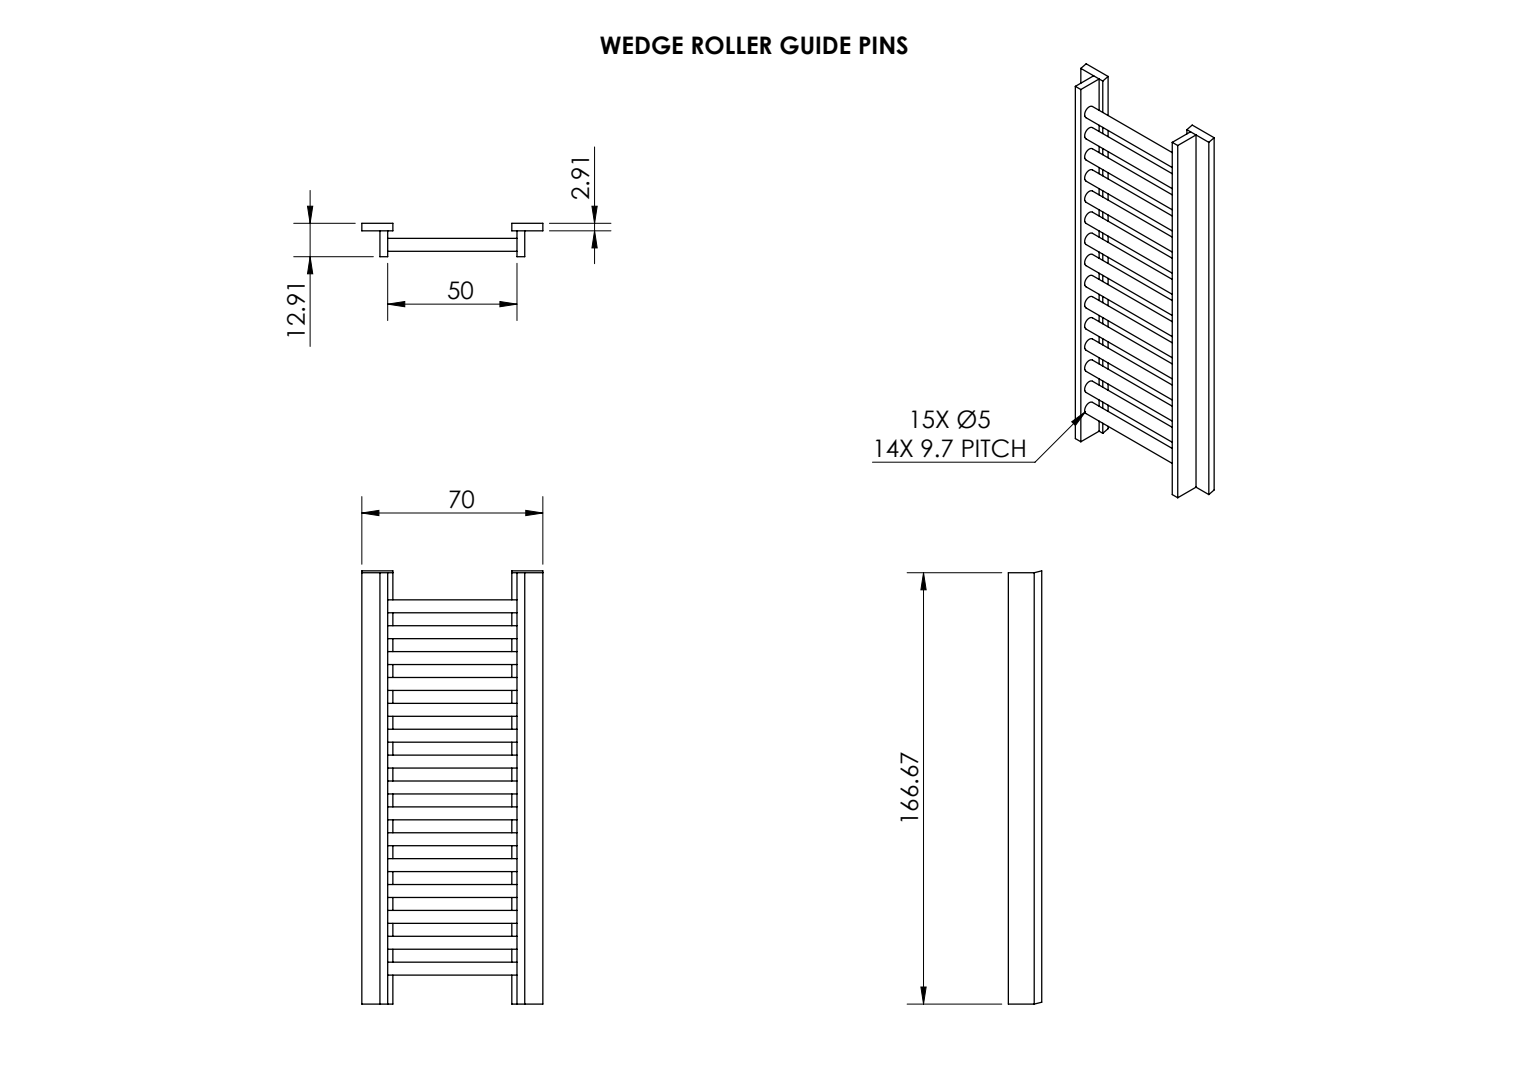
ISO-10303-21;
HEADER;
FILE_DESCRIPTION (('STEP AP214'),
    '1' );
FILE_NAME ('Wedge Roller Guide Pins.step',
    '2026-09-24T10:26:00',
    ( '' ),
    ( '' ),
    'SwSTEP 2.0',
    'SolidWorks 2026',
    '' );
FILE_SCHEMA (( 'AUTOMOTIVE_DESIGN' ));
ENDSEC;

DATA;
#3=CARTESIAN_POINT ( 'NONE',  ( 34.85300976710104948, 100.8957249956400375, 25.00000000000000000 ) ) ;
#7=CARTESIAN_POINT ( 'NONE',  ( 59.10657227073432551, 3.881474981106830313, 25.00000000000000000 ) ) ;
#45=VERTEX_POINT ( 'NONE', #1089 ) ;
#50=CIRCLE ( 'NONE', #10087, 2.500000000000002220 ) ;
#51=CIRCLE ( 'NONE', #7981, 2.500000000000002220 ) ;
#55=VERTEX_POINT ( 'NONE', #5546 ) ;
#59=MECHANICAL_DESIGN_GEOMETRIC_PRESENTATION_REPRESENTATION('',(#3339),#8217);
#68=DIRECTION ( 'NONE',  ( -1.000000000000000000, 0.000000000000000000, 0.000000000000000000 ) ) ;
#75=EDGE_CURVE ( 'NONE', #7740, #14384, #13409, .T. ) ;
#106=LINE ( 'NONE', #11351, #1126 ) ;
#108=( NAMED_UNIT ( * ) PLANE_ANGLE_UNIT ( ) SI_UNIT ( $, .RADIAN. ) );
#114=CYLINDRICAL_SURFACE ( 'NONE', #8701, 2.500000000000002220 ) ;
#138=AXIS2_PLACEMENT_3D ( 'NONE', #9240, #11510, #4853 ) ;
#139=FACE_OUTER_BOUND ( 'NONE', #10085, .T. ) ;
#141=EDGE_CURVE ( 'NONE', #4176, #9400, #11330, .T. ) ;
#150=EDGE_CURVE ( 'NONE', #7089, #2949, #9184, .T. ) ;
#158=ORIENTED_EDGE ( 'NONE', *, *, #2244, .F. ) ;
#159=CARTESIAN_POINT ( 'NONE',  ( 56.68121602037099649, 13.58289998256015352, 25.00000000000000000 ) ) ;
#167=CARTESIAN_POINT ( 'NONE',  ( 0.000000000000000000, 0.000000000000000000, 0.000000000000000000 ) ) ;
#174=LINE ( 'NONE', #1203, #523 ) ;
#175=AXIS2_PLACEMENT_3D ( 'NONE', #2230, #7697, #10922 ) ;
#184=DIRECTION ( 'NONE',  ( -1.000000000000000000, 0.000000000000000000, 0.000000000000000000 ) ) ;
#187=AXIS2_PLACEMENT_3D ( 'NONE', #14289, #6433, #6375 ) ;
#192=VERTEX_POINT ( 'NONE', #361 ) ;
#207=ORIENTED_EDGE ( 'NONE', *, *, #6472, .T. ) ;
#217=CARTESIAN_POINT ( 'NONE',  ( 56.75585977000769589, 23.28432498401347672, 25.00000000000000000 ) ) ;
#219=CARTESIAN_POINT ( 'NONE',  ( 62.10586122665984732, -20.42344490663941414, -23.00000000000000000 ) ) ;
#245=ORIENTED_EDGE ( 'NONE', *, *, #3357, .T. ) ;
#255=DIRECTION ( 'NONE',  ( 0.000000000000000000, 0.000000000000000000, 1.000000000000000000 ) ) ;
#257=FACE_OUTER_BOUND ( 'NONE', #7644, .T. ) ;
#260=VERTEX_POINT ( 'NONE', #11845 ) ;
#262=VECTOR ( 'NONE', #2943, 1000.000000000000114 ) ;
#271=CARTESIAN_POINT ( 'NONE',  ( 66.53192852109765454, -5.819950020346492892, -25.00000000000000000 ) ) ;
#280=CYLINDRICAL_SURFACE ( 'NONE', #1408, 2.500000000000002220 ) ;
#290=DIRECTION ( 'NONE',  ( -1.000000000000000000, 0.000000000000000000, 0.000000000000000000 ) ) ;
#293=EDGE_CURVE ( 'NONE', #3067, #10101, #2628, .T. ) ;
#296=CARTESIAN_POINT ( 'NONE',  ( 61.53192852109764743, -5.819950020346492892, -25.00000000000000000 ) ) ;
#304=CARTESIAN_POINT ( 'NONE',  ( 63.34848382498275754, 15.83712095624566984, 0.000000000000000000 ) ) ;
#318=DIRECTION ( 'NONE',  ( 0.000000000000000000, 0.000000000000000000, -1.000000000000000000 ) ) ;
#319=AXIS2_PLACEMENT_3D ( 'NONE', #14262, #4250, #9862 ) ;
#332=EDGE_LOOP ( 'NONE', ( #2235, #9839 ) ) ;
#356=EDGE_CURVE ( 'NONE', #7502, #4025, #7084, .T. ) ;
#361=CARTESIAN_POINT ( 'NONE',  ( 35.00229726637439143, 120.2985749985466839, 25.00000000000000000 ) ) ;
#367=EDGE_CURVE ( 'NONE', #6880, #5464, #10123, .T. ) ;
#370=ADVANCED_FACE ( 'NONE', ( #3209 ), #923, .F. ) ;
#385=CARTESIAN_POINT ( 'NONE',  ( 54.33050351964436686, 32.98574998546678927, 25.00000000000000000 ) ) ;
#403=ORIENTED_EDGE ( 'NONE', *, *, #3357, .F. ) ;
#418=EDGE_CURVE ( 'NONE', #12547, #7049, #5258, .T. ) ;
#436=VECTOR ( 'NONE', #12555, 999.9999999999998863 ) ;
#450=ORIENTED_EDGE ( 'NONE', *, *, #2914, .T. ) ;
#453=DIRECTION ( 'NONE',  ( 0.000000000000000000, 0.000000000000000000, -1.000000000000000000 ) ) ;
#461=CARTESIAN_POINT ( 'NONE',  ( 63.34848382498275754, 15.83712095624566984, 0.000000000000000000 ) ) ;
#474=ORIENTED_EDGE ( 'NONE', *, *, #4676, .T. ) ;
#482=PLANE ( 'NONE',  #7880 ) ;
#483=DIRECTION ( 'NONE',  ( 0.000000000000000000, 0.000000000000000000, -1.000000000000000000 ) ) ;
#490=DIRECTION ( 'NONE',  ( 1.000000000000000000, 0.000000000000000000, 0.000000000000000000 ) ) ;
#494=CARTESIAN_POINT ( 'NONE',  ( 49.55443476855437268, 62.09002498982675888, 25.00000000000000000 ) ) ;
#516=ORIENTED_EDGE ( 'NONE', *, *, #14434, .F. ) ;
#523=VECTOR ( 'NONE', #2168, 1000.000000000000000 ) ;
#536=CARTESIAN_POINT ( 'NONE',  ( 37.35300976710104948, 100.8957249956400375, -25.00000000000000000 ) ) ;
#544=LINE ( 'NONE', #5067, #7395 ) ;
#552=APPLICATION_CONTEXT ( 'automotive_design' ) ;
#554=AXIS2_PLACEMENT_3D ( 'NONE', #7102, #318, #1552 ) ;
#556=EDGE_CURVE ( 'NONE', #7883, #4518, #5673, .T. ) ;
#558=ORIENTED_EDGE ( 'NONE', *, *, #7367, .T. ) ;
#561=AXIS2_PLACEMENT_3D ( 'NONE', #10302, #7885, #290 ) ;
#563=CARTESIAN_POINT ( 'NONE',  ( 61.60657227073433262, 3.881474981106830313, 25.00000000000000000 ) ) ;
#564=FACE_BOUND ( 'NONE', #13096, .T. ) ;
#566=DIRECTION ( 'NONE',  ( 0.000000000000000000, 0.000000000000000000, 1.000000000000000000 ) ) ;
#581=CARTESIAN_POINT ( 'NONE',  ( 0.000000000000000000, 0.000000000000000000, 35.00000000000000000 ) ) ;
#591=CARTESIAN_POINT ( 'NONE',  ( 30.00229726637438432, 120.2985749985466839, -25.00000000000000000 ) ) ;
#596=DIRECTION ( 'NONE',  ( -1.000000000000000000, 0.000000000000000000, 0.000000000000000000 ) ) ;
#614=CARTESIAN_POINT ( 'NONE',  ( 54.25585977000769589, 23.28432498401347672, 25.00000000000000000 ) ) ;
#635=DIRECTION ( 'NONE',  ( 0.000000000000000000, 0.000000000000000000, 1.000000000000000000 ) ) ;
#648=DIRECTION ( 'NONE',  ( 0.000000000000000000, 0.000000000000000000, -1.000000000000000000 ) ) ;
#666=AXIS2_PLACEMENT_3D ( 'NONE', #7553, #831, #14236 ) ;
#674=EDGE_CURVE ( 'NONE', #2739, #5618, #12700, .T. ) ;
#677=VECTOR ( 'NONE', #3560, 999.9999999999998863 ) ;
#680=ORIENTED_EDGE ( 'NONE', *, *, #3167, .T. ) ;
#684=CARTESIAN_POINT ( 'NONE',  ( 62.10586122665984732, -20.42344490663941414, 35.00000000000000000 ) ) ;
#685=EDGE_CURVE ( 'NONE', #3184, #7164, #14140, .T. ) ;
#689=CARTESIAN_POINT ( 'NONE',  ( 64.03192852109765454, -5.819950020346492892, 25.00000000000000000 ) ) ;
#696=VERTEX_POINT ( 'NONE', #8297 ) ;
#707=FACE_BOUND ( 'NONE', #8200, .T. ) ;
#727=DIRECTION ( 'NONE',  ( -0.9701425001453319874, -0.2425356250363328026, 0.000000000000000000 ) ) ;
#729=DIRECTION ( 'NONE',  ( 0.000000000000000000, 0.000000000000000000, -1.000000000000000000 ) ) ;
#778=CARTESIAN_POINT ( 'NONE',  ( 71.80728622811317052, -17.99808865627607801, 28.00000000000000000 ) ) ;
#788=PLANE ( 'NONE',  #1131 ) ;
#793=CYLINDRICAL_SURFACE ( 'NONE', #14229, 2.500000000000002220 ) ;
#812=LINE ( 'NONE', #2952, #993 ) ;
#828=CARTESIAN_POINT ( 'NONE',  ( 51.90514726928103073, 42.68717498692012668, 25.00000000000000000 ) ) ;
#829=ORIENTED_EDGE ( 'NONE', *, *, #5080, .F. ) ;
#830=ORIENTED_EDGE ( 'NONE', *, *, #13086, .T. ) ;
#831=DIRECTION ( 'NONE',  ( 0.000000000000000000, 0.000000000000000000, -1.000000000000000000 ) ) ;
#833=ORIENTED_EDGE ( 'NONE', *, *, #2397, .F. ) ;
#848=DIRECTION ( 'NONE',  ( -1.000000000000000000, 0.000000000000000000, 0.000000000000000000 ) ) ;
#852=SHAPE_REPRESENTATION ( 'Wedge Roller Guide Pins', ( #11025 ), #12660 ) ;
#861=DIRECTION ( 'NONE',  ( 0.000000000000000000, 0.000000000000000000, -1.000000000000000000 ) ) ;
#877=ORIENTED_EDGE ( 'NONE', *, *, #367, .F. ) ;
#884=CIRCLE ( 'NONE', #1928, 2.500000000000002220 ) ;
#896=CARTESIAN_POINT ( 'NONE',  ( 66.53192852109765454, -5.819950020346492892, 25.00000000000000000 ) ) ;
#899=ORIENTED_EDGE ( 'NONE', *, *, #1154, .F. ) ;
#901=FACE_BOUND ( 'NONE', #9182, .T. ) ;
#903=EDGE_LOOP ( 'NONE', ( #2586, #3281, #10639, #10466 ) ) ;
#908=VERTEX_POINT ( 'NONE', #4230 ) ;
#911=CARTESIAN_POINT ( 'NONE',  ( 61.60657227073433262, 3.881474981106830313, 25.00000000000000000 ) ) ;
#921=ORIENTED_EDGE ( 'NONE', *, *, #4211, .T. ) ;
#922=VECTOR ( 'NONE', #9203, 1000.000000000000114 ) ;
#923=PLANE ( 'NONE',  #8498 ) ;
#945=VECTOR ( 'NONE', #3041, 1000.000000000000000 ) ;
#952=CARTESIAN_POINT ( 'NONE',  ( 47.05443476855437268, 62.09002498982675888, 25.00000000000000000 ) ) ;
#956=DIRECTION ( 'NONE',  ( 1.000000000000000000, 0.000000000000000000, 0.000000000000000000 ) ) ;
#958=DIRECTION ( 'NONE',  ( 0.000000000000000000, 0.000000000000000000, -1.000000000000000000 ) ) ;
#971=ORIENTED_EDGE ( 'NONE', *, *, #11807, .T. ) ;
#979=AXIS2_PLACEMENT_3D ( 'NONE', #13212, #11893, #4294 ) ;
#992=VERTEX_POINT ( 'NONE', #4519 ) ;
#993=VECTOR ( 'NONE', #12897, 999.9999999999998863 ) ;
#1038=CARTESIAN_POINT ( 'NONE',  ( 18.68170757442808849, 141.2731697022877313, 35.00000000000000000 ) ) ;
#1050=CARTESIAN_POINT ( 'NONE',  ( 31.38313257588138683, 143.6985259526510390, -28.00000000000000000 ) ) ;
#1054=PRESENTATION_STYLE_ASSIGNMENT (( #2158 ) ) ;
#1055=EDGE_LOOP ( 'NONE', ( #1751, #5944 ) ) ;
#1058=DIRECTION ( 'NONE',  ( -1.000000000000000000, 0.000000000000000000, 0.000000000000000000 ) ) ;
#1087=ORIENTED_EDGE ( 'NONE', *, *, #7522, .T. ) ;
#1089=CARTESIAN_POINT ( 'NONE',  ( 62.10586122665987574, -20.42344490663940704, -28.00000000000000000 ) ) ;
#1090=ORIENTED_EDGE ( 'NONE', *, *, #9852, .F. ) ;
#1094=CARTESIAN_POINT ( 'NONE',  ( 27.57694101601105530, 130.0000000000000000, 25.00000000000000000 ) ) ;
#1095=CARTESIAN_POINT ( 'NONE',  ( 42.20372226782770753, 81.49287499273339108, 25.00000000000000000 ) ) ;
#1112=FACE_OUTER_BOUND ( 'NONE', #2519, .T. ) ;
#1114=CARTESIAN_POINT ( 'NONE',  ( 47.05443476855437268, 62.09002498982675888, 25.00000000000000000 ) ) ;
#1121=CARTESIAN_POINT ( 'NONE',  ( 54.40514726928103784, 42.68717498692012668, 25.00000000000000000 ) ) ;
#1125=LINE ( 'NONE', #8872, #7058 ) ;
#1126=VECTOR ( 'NONE', #6747, 1000.000000000000000 ) ;
#1131=AXIS2_PLACEMENT_3D ( 'NONE', #7566, #1881, #14324 ) ;
#1147=EDGE_LOOP ( 'NONE', ( #6680, #4247, #9054, #1407 ) ) ;
#1149=ORIENTED_EDGE ( 'NONE', *, *, #1431, .F. ) ;
#1154=EDGE_CURVE ( 'NONE', #13574, #3245, #13934, .T. ) ;
#1159=AXIS2_PLACEMENT_3D ( 'NONE', #13106, #727, #3082 ) ;
#1176=VERTEX_POINT ( 'NONE', #5217 ) ;
#1180=DIRECTION ( 'NONE',  ( 0.000000000000000000, 0.000000000000000000, -1.000000000000000000 ) ) ;
#1193=DIRECTION ( 'NONE',  ( -0.000000000000000000, -0.000000000000000000, -1.000000000000000000 ) ) ;
#1195=ORIENTED_EDGE ( 'NONE', *, *, #13325, .F. ) ;
#1197=ORIENTED_EDGE ( 'NONE', *, *, #11455, .F. ) ;
#1198=EDGE_CURVE ( 'NONE', #11002, #6663, #1854, .T. ) ;
#1199=CIRCLE ( 'NONE', #6095, 2.500000000000002220 ) ;
#1203=CARTESIAN_POINT ( 'NONE',  ( 44.70372226782771463, 81.49287499273339108, 25.00000000000000000 ) ) ;
#1207=DIRECTION ( 'NONE',  ( 0.000000000000000000, 0.000000000000000000, -1.000000000000000000 ) ) ;
#1208=ORIENTED_EDGE ( 'NONE', *, *, #13188, .T. ) ;
#1210=VERTEX_POINT ( 'NONE', #11953 ) ;
#1218=ADVANCED_FACE ( 'NONE', ( #8573 ), #10705, .T. ) ;
#1221=ORIENTED_EDGE ( 'NONE', *, *, #3777, .T. ) ;
#1242=VECTOR ( 'NONE', #3558, 1000.000000000000000 ) ;
#1251=ORIENTED_EDGE ( 'NONE', *, *, #10457, .T. ) ;
#1266=EDGE_CURVE ( 'NONE', #9400, #6663, #2842, .T. ) ;
#1275=CARTESIAN_POINT ( 'NONE',  ( 42.20372226782770753, 81.49287499273339108, 25.00000000000000000 ) ) ;
#1280=ORIENTED_EDGE ( 'NONE', *, *, #13856, .T. ) ;
#1292=CYLINDRICAL_SURFACE ( 'NONE', #4914, 2.500000000000002220 ) ;
#1300=CARTESIAN_POINT ( 'NONE',  ( 56.68121602037099649, 13.58289998256015352, 25.00000000000000000 ) ) ;
#1312=DIRECTION ( 'NONE',  ( -0.000000000000000000, -0.000000000000000000, -1.000000000000000000 ) ) ;
#1328=VERTEX_POINT ( 'NONE', #7687 ) ;
#1349=AXIS2_PLACEMENT_3D ( 'NONE', #1038, #4350, #9963 ) ;
#1351=AXIS2_PLACEMENT_3D ( 'NONE', #12401, #11364, #7926 ) ;
#1378=LINE ( 'NONE', #10313, #262 ) ;
#1385=ORIENTED_EDGE ( 'NONE', *, *, #13324, .T. ) ;
#1389=AXIS2_PLACEMENT_3D ( 'NONE', #2479, #13763, #7222 ) ;
#1407=ORIENTED_EDGE ( 'NONE', *, *, #10352, .T. ) ;
#1408=AXIS2_PLACEMENT_3D ( 'NONE', #4546, #5891, #4746 ) ;
#1409=DIRECTION ( 'NONE',  ( 0.000000000000000000, 0.000000000000000000, 1.000000000000000000 ) ) ;
#1421=CARTESIAN_POINT ( 'NONE',  ( 21.68170757442808849, 141.2731697022877313, 35.00000000000000000 ) ) ;
#1425=AXIS2_PLACEMENT_3D ( 'NONE', #7083, #3889, #12576 ) ;
#1431=EDGE_CURVE ( 'NONE', #4518, #7883, #10070, .T. ) ;
#1439=AXIS2_PLACEMENT_3D ( 'NONE', #11177, #2196, #10158 ) ;
#1449=AXIS2_PLACEMENT_3D ( 'NONE', #4221, #13074, #9757 ) ;
#1452=ORIENTED_EDGE ( 'NONE', *, *, #11500, .F. ) ;
#1453=EDGE_CURVE ( 'NONE', #7600, #3428, #1733, .T. ) ;
#1457=CARTESIAN_POINT ( 'NONE',  ( 37.27836601746437850, 91.19429999418670718, 25.00000000000000000 ) ) ;
#1459=ADVANCED_FACE ( 'NONE', ( #12163 ), #10983, .T. ) ;
#1480=FACE_OUTER_BOUND ( 'NONE', #4601, .T. ) ;
#1481=ADVANCED_FACE ( 'NONE', ( #1112 ), #5566, .T. ) ;
#1484=VERTEX_POINT ( 'NONE', #11203 ) ;
#1508=ORIENTED_EDGE ( 'NONE', *, *, #9688, .F. ) ;
#1532=CARTESIAN_POINT ( 'NONE',  ( 51.90514726928103073, 42.68717498692012668, 25.00000000000000000 ) ) ;
#1549=PLANE ( 'NONE',  #5866 ) ;
#1552=DIRECTION ( 'NONE',  ( -1.000000000000000000, 0.000000000000000000, 0.000000000000000000 ) ) ;
#1567=ORIENTED_EDGE ( 'NONE', *, *, #556, .T. ) ;
#1569=FACE_BOUND ( 'NONE', #11379, .T. ) ;
#1576=ADVANCED_FACE ( 'NONE', ( #4836 ), #8046, .T. ) ;
#1587=AXIS2_PLACEMENT_3D ( 'NONE', #581, #9640, #10739 ) ;
#1595=AXIS2_PLACEMENT_3D ( 'NONE', #2769, #12950, #6194 ) ;
#1609=ORIENTED_EDGE ( 'NONE', *, *, #9227, .F. ) ;
#1638=DIRECTION ( 'NONE',  ( -1.000000000000000000, 0.000000000000000000, 0.000000000000000000 ) ) ;
#1640=LINE ( 'NONE', #6011, #3763 ) ;
#1646=LINE ( 'NONE', #778, #12787 ) ;
#1648=FACE_BOUND ( 'NONE', #6730, .T. ) ;
#1676=LINE ( 'NONE', #2631, #9345 ) ;
#1679=LINE ( 'NONE', #7224, #8428 ) ;
#1689=VECTOR ( 'NONE', #13552, 1000.000000000000000 ) ;
#1700=CIRCLE ( 'NONE', #7988, 2.500000000000002220 ) ;
#1702=VERTEX_POINT ( 'NONE', #11867 ) ;
#1703=ORIENTED_EDGE ( 'NONE', *, *, #2205, .F. ) ;
#1719=DIRECTION ( 'NONE',  ( 0.000000000000000000, 0.000000000000000000, 1.000000000000000000 ) ) ;
#1725=PLANE ( 'NONE',  #4726 ) ;
#1733=LINE ( 'NONE', #10655, #7488 ) ;
#1735=ORIENTED_EDGE ( 'NONE', *, *, #13842, .F. ) ;
#1751=ORIENTED_EDGE ( 'NONE', *, *, #13733, .F. ) ;
#1781=VERTEX_POINT ( 'NONE', #10624 ) ;
#1786=CARTESIAN_POINT ( 'NONE',  ( 44.70372226782771463, 81.49287499273339108, -25.00000000000000000 ) ) ;
#1789=CARTESIAN_POINT ( 'NONE',  ( 21.68170757442808849, 141.2731697022877313, -35.00000000000000000 ) ) ;
#1801=FACE_OUTER_BOUND ( 'NONE', #11405, .T. ) ;
#1813=AXIS2_PLACEMENT_3D ( 'NONE', #8430, #7399, #9537 ) ;
#1819=EDGE_CURVE ( 'NONE', #4025, #7502, #11428, .T. ) ;
#1842=CARTESIAN_POINT ( 'NONE',  ( 62.10586122665984732, -20.42344490663941414, -35.00000000000000000 ) ) ;
#1846=EDGE_LOOP ( 'NONE', ( #9526, #2877, #13120, #11097 ) ) ;
#1849=DIRECTION ( 'NONE',  ( 1.000000000000000000, 0.000000000000000000, 0.000000000000000000 ) ) ;
#1851=EDGE_CURVE ( 'NONE', #8043, #3245, #6575, .T. ) ;
#1854=LINE ( 'NONE', #10984, #945 ) ;
#1881=DIRECTION ( 'NONE',  ( 0.9701425001453319874, 0.2425356250363328026, 0.000000000000000000 ) ) ;
#1897=CARTESIAN_POINT ( 'NONE',  ( 31.38313257588138683, 143.6985259526510390, -28.00000000000000000 ) ) ;
#1911=ADVANCED_FACE ( 'NONE', ( #13331 ), #6651, .T. ) ;
#1917=DIRECTION ( 'NONE',  ( 0.000000000000000000, 0.000000000000000000, -1.000000000000000000 ) ) ;
#1925=FACE_OUTER_BOUND ( 'NONE', #13791, .T. ) ;
#1928=AXIS2_PLACEMENT_3D ( 'NONE', #11960, #10917, #1936 ) ;
#1931=CARTESIAN_POINT ( 'NONE',  ( 59.18121602037099649, 13.58289998256015352, -25.00000000000000000 ) ) ;
#1932=CARTESIAN_POINT ( 'NONE',  ( 54.25585977000769589, 23.28432498401347672, 25.00000000000000000 ) ) ;
#1935=CARTESIAN_POINT ( 'NONE',  ( 21.68170757442808849, 141.2731697022877313, -28.00000000000000000 ) ) ;
#1936=DIRECTION ( 'NONE',  ( -1.000000000000000000, 0.000000000000000000, 0.000000000000000000 ) ) ;
#1949=ORIENTED_EDGE ( 'NONE', *, *, #5722, .F. ) ;
#1967=AXIS2_PLACEMENT_3D ( 'NONE', #4821, #13841, #8319 ) ;
#1972=ORIENTED_EDGE ( 'NONE', *, *, #2543, .T. ) ;
#1976=LINE ( 'NONE', #4258, #14222 ) ;
#1985=VERTEX_POINT ( 'NONE', #296 ) ;
#1991=CARTESIAN_POINT ( 'NONE',  ( 44.62907851819101523, 71.79144999128007498, 25.00000000000000000 ) ) ;
#2001=FACE_OUTER_BOUND ( 'NONE', #12684, .T. ) ;
#2007=EDGE_LOOP ( 'NONE', ( #10274, #2455, #12573, #207 ) ) ;
#2024=CYLINDRICAL_SURFACE ( 'NONE', #7905, 2.500000000000002220 ) ;
#2028=ORIENTED_EDGE ( 'NONE', *, *, #1154, .T. ) ;
#2031=ORIENTED_EDGE ( 'NONE', *, *, #4339, .T. ) ;
#2033=VERTEX_POINT ( 'NONE', #9434 ) ;
#2039=LINE ( 'NONE', #7733, #7005 ) ;
#2045=ORIENTED_EDGE ( 'NONE', *, *, #5645, .T. ) ;
#2046=CARTESIAN_POINT ( 'NONE',  ( 46.97979101891770171, 52.38859998837343568, 25.00000000000000000 ) ) ;
#2104=ORIENTED_EDGE ( 'NONE', *, *, #7153, .F. ) ;
#2107=VERTEX_POINT ( 'NONE', #9509 ) ;
#2108=DIRECTION ( 'NONE',  ( 0.000000000000000000, 0.000000000000000000, -1.000000000000000000 ) ) ;
#2110=CARTESIAN_POINT ( 'NONE',  ( 61.68121602037100359, 13.58289998256015352, -25.00000000000000000 ) ) ;
#2112=DIRECTION ( 'NONE',  ( 0.000000000000000000, 0.000000000000000000, -1.000000000000000000 ) ) ;
#2117=CIRCLE ( 'NONE', #12161, 2.500000000000002220 ) ;
#2132=LINE ( 'NONE', #6724, #14200 ) ;
#2146=CARTESIAN_POINT ( 'NONE',  ( 51.90514726928103073, 42.68717498692012668, 25.00000000000000000 ) ) ;
#2151=CIRCLE ( 'NONE', #10317, 2.500000000000002220 ) ;
#2158=SURFACE_STYLE_USAGE ( .BOTH. , #3257 ) ;
#2163=DIRECTION ( 'NONE',  ( 1.000000000000000000, 0.000000000000000000, 0.000000000000000000 ) ) ;
#2168=DIRECTION ( 'NONE',  ( 0.000000000000000000, 0.000000000000000000, -1.000000000000000000 ) ) ;
#2173=AXIS2_PLACEMENT_3D ( 'NONE', #3670, #3744, #4828 ) ;
#2185=ORIENTED_EDGE ( 'NONE', *, *, #3297, .F. ) ;
#2191=FACE_OUTER_BOUND ( 'NONE', #4724, .T. ) ;
#2193=DIRECTION ( 'NONE',  ( -1.000000000000000000, 0.000000000000000000, 0.000000000000000000 ) ) ;
#2196=DIRECTION ( 'NONE',  ( 0.000000000000000000, 0.000000000000000000, -1.000000000000000000 ) ) ;
#2205=EDGE_CURVE ( 'NONE', #4466, #1781, #5262, .T. ) ;
#2206=EDGE_LOOP ( 'NONE', ( #1087, #5917 ) ) ;
#2211=CARTESIAN_POINT ( 'NONE',  ( 18.68170757442808849, 141.2731697022877313, 23.00000000000000000 ) ) ;
#2224=CARTESIAN_POINT ( 'NONE',  ( 64.10657227073433262, 3.881474981106830757, 25.00000000000000000 ) ) ;
#2230=CARTESIAN_POINT ( 'NONE',  ( 56.75585977000769589, 23.28432498401347672, -25.00000000000000000 ) ) ;
#2235=ORIENTED_EDGE ( 'NONE', *, *, #13324, .F. ) ;
#2237=CARTESIAN_POINT ( 'NONE',  ( 51.97979101891770171, 52.38859998837343568, -25.00000000000000000 ) ) ;
#2244=EDGE_CURVE ( 'NONE', #10101, #9931, #10957, .T. ) ;
#2246=PRESENTATION_STYLE_ASSIGNMENT (( #13299 ) ) ;
#2257=CARTESIAN_POINT ( 'NONE',  ( 71.80728622811317052, -17.99808865627607801, -25.00000000000000000 ) ) ;
#2259=FACE_OUTER_BOUND ( 'NONE', #11276, .T. ) ;
#2274=DIRECTION ( 'NONE',  ( 0.000000000000000000, 0.000000000000000000, -1.000000000000000000 ) ) ;
#2279=ADVANCED_FACE ( 'NONE', ( #7729 ), #9722, .T. ) ;
#2297=ORIENTED_EDGE ( 'NONE', *, *, #7367, .F. ) ;
#2302=CARTESIAN_POINT ( 'NONE',  ( 35.00229726637439143, 120.2985749985466839, -25.00000000000000000 ) ) ;
#2318=DIRECTION ( 'NONE',  ( 0.000000000000000000, 0.000000000000000000, 1.000000000000000000 ) ) ;
#2330=CARTESIAN_POINT ( 'NONE',  ( 71.80728622811317052, -17.99808865627607801, -25.00000000000000000 ) ) ;
#2332=ORIENTED_EDGE ( 'NONE', *, *, #7478, .T. ) ;
#2348=EDGE_CURVE ( 'NONE', #8916, #9931, #10213, .T. ) ;
#2355=AXIS2_PLACEMENT_3D ( 'NONE', #2146, #958, #12091 ) ;
#2368=( LENGTH_UNIT ( ) NAMED_UNIT ( * ) SI_UNIT ( .MILLI., .METRE. ) );
#2370=CARTESIAN_POINT ( 'NONE',  ( 64.10657227073433262, 3.881474981106830757, -25.00000000000000000 ) ) ;
#2373=VECTOR ( 'NONE', #5556, 1000.000000000000000 ) ;
#2380=DIRECTION ( 'NONE',  ( -0.000000000000000000, -0.000000000000000000, -1.000000000000000000 ) ) ;
#2382=LINE ( 'NONE', #12536, #10066 ) ;
#2392=EDGE_CURVE ( 'NONE', #11916, #5464, #3580, .T. ) ;
#2393=EDGE_LOOP ( 'NONE', ( #9202, #2609, #2185, #9680 ) ) ;
#2397=EDGE_CURVE ( 'NONE', #260, #5200, #8016, .T. ) ;
#2399=DIRECTION ( 'NONE',  ( 1.000000000000000000, 0.000000000000000000, 0.000000000000000000 ) ) ;
#2417=DIRECTION ( 'NONE',  ( 0.000000000000000000, 0.000000000000000000, -1.000000000000000000 ) ) ;
#2428=CYLINDRICAL_SURFACE ( 'NONE', #13729, 2.500000000000002220 ) ;
#2446=SHAPE_REPRESENTATION_RELATIONSHIP ( 'NONE' , 'NONE' ,  #852, #6268 ) ;
#2447=DIRECTION ( 'NONE',  ( -1.000000000000000000, 0.000000000000000000, 0.000000000000000000 ) ) ;
#2455=ORIENTED_EDGE ( 'NONE', *, *, #12096, .F. ) ;
#2458=ADVANCED_FACE ( 'NONE', ( #11171 ), #6259, .T. ) ;
#2460=VECTOR ( 'NONE', #13939, 1000.000000000000000 ) ;
#2473=VECTOR ( 'NONE', #2726, 1000.000000000000114 ) ;
#2479=CARTESIAN_POINT ( 'NONE',  ( 44.62907851819101523, 71.79144999128007498, -25.00000000000000000 ) ) ;
#2491=AXIS2_PLACEMENT_3D ( 'NONE', #8792, #9971, #5638 ) ;
#2497=ORIENTED_EDGE ( 'NONE', *, *, #9688, .T. ) ;
#2503=EDGE_CURVE ( 'NONE', #2898, #7089, #7209, .T. ) ;
#2505=FACE_OUTER_BOUND ( 'NONE', #5939, .T. ) ;
#2513=CARTESIAN_POINT ( 'NONE',  ( 0.000000000000000000, 0.000000000000000000, -23.00000000000000000 ) ) ;
#2517=EDGE_CURVE ( 'NONE', #4300, #2898, #12321, .T. ) ;
#2519=EDGE_LOOP ( 'NONE', ( #13497, #2819, #2761, #13622 ) ) ;
#2520=DIRECTION ( 'NONE',  ( 0.000000000000000000, 0.000000000000000000, -1.000000000000000000 ) ) ;
#2522=DIRECTION ( 'NONE',  ( 0.000000000000000000, 0.000000000000000000, -1.000000000000000000 ) ) ;
#2539=DIRECTION ( 'NONE',  ( -0.000000000000000000, -0.000000000000000000, -1.000000000000000000 ) ) ;
#2540=DIRECTION ( 'NONE',  ( 0.000000000000000000, 0.000000000000000000, -1.000000000000000000 ) ) ;
#2542=DIRECTION ( 'NONE',  ( 1.000000000000000000, 0.000000000000000000, 0.000000000000000000 ) ) ;
#2543=EDGE_CURVE ( 'NONE', #3708, #1484, #11614, .T. ) ;
#2553=ORIENTED_EDGE ( 'NONE', *, *, #356, .F. ) ;
#2557=DIRECTION ( 'NONE',  ( 0.000000000000000000, 0.000000000000000000, -1.000000000000000000 ) ) ;
#2563=FACE_OUTER_BOUND ( 'NONE', #3025, .T. ) ;
#2571=CARTESIAN_POINT ( 'NONE',  ( 59.10586122665984732, -20.42344490663941414, 23.00000000000000000 ) ) ;
#2586=ORIENTED_EDGE ( 'NONE', *, *, #5645, .F. ) ;
#2589=MECHANICAL_DESIGN_GEOMETRIC_PRESENTATION_REPRESENTATION('',(#8435),#6081);
#2598=ORIENTED_EDGE ( 'NONE', *, *, #13375, .T. ) ;
#2602=CIRCLE ( 'NONE', #5843, 2.500000000000002220 ) ;
#2603=VERTEX_POINT ( 'NONE', #13163 ) ;
#2609=ORIENTED_EDGE ( 'NONE', *, *, #4181, .F. ) ;
#2627=ORIENTED_EDGE ( 'NONE', *, *, #685, .T. ) ;
#2628=LINE ( 'NONE', #9428, #14127 ) ;
#2631=CARTESIAN_POINT ( 'NONE',  ( 59.10586122665984732, -20.42344490663941414, -35.00000000000000000 ) ) ;
#2633=LINE ( 'NONE', #13548, #9880 ) ;
#2644=LINE ( 'NONE', #13638, #12931 ) ;
#2651=DIRECTION ( 'NONE',  ( 0.000000000000000000, 0.000000000000000000, -1.000000000000000000 ) ) ;
#2656=DIRECTION ( 'NONE',  ( 0.000000000000000000, 0.000000000000000000, -1.000000000000000000 ) ) ;
#2664=ORIENTED_EDGE ( 'NONE', *, *, #11015, .F. ) ;
#2673=VERTEX_POINT ( 'NONE', #7491 ) ;
#2676=ORIENTED_EDGE ( 'NONE', *, *, #6472, .F. ) ;
#2683=ADVANCED_FACE ( 'NONE', ( #13297 ), #788, .F. ) ;
#2693=CARTESIAN_POINT ( 'NONE',  ( 56.75585977000769589, 23.28432498401347672, 25.00000000000000000 ) ) ;
#2695=DIRECTION ( 'NONE',  ( -1.000000000000000000, 0.000000000000000000, 0.000000000000000000 ) ) ;
#2718=ADVANCED_FACE ( 'NONE', ( #9771 ), #10939, .T. ) ;
#2720=CARTESIAN_POINT ( 'NONE',  ( 31.38313257588138683, 143.6985259526510390, 28.00000000000000000 ) ) ;
#2726=DIRECTION ( 'NONE',  ( -0.9701425001453318764, -0.2425356250363329969, 0.000000000000000000 ) ) ;
#2729=EDGE_CURVE ( 'NONE', #3826, #3362, #6267, .T. ) ;
#2737=LINE ( 'NONE', #4849, #1242 ) ;
#2738=DIRECTION ( 'NONE',  ( 0.000000000000000000, 0.000000000000000000, -1.000000000000000000 ) ) ;
#2739=VERTEX_POINT ( 'NONE', #6688 ) ;
#2750=VECTOR ( 'NONE', #2540, 1000.000000000000000 ) ;
#2756=FACE_BOUND ( 'NONE', #2206, .T. ) ;
#2761=ORIENTED_EDGE ( 'NONE', *, *, #3247, .F. ) ;
#2769=CARTESIAN_POINT ( 'NONE',  ( 54.33050351964436686, 32.98574998546678927, 25.00000000000000000 ) ) ;
#2772=CARTESIAN_POINT ( 'NONE',  ( 56.75585977000769589, 23.28432498401347672, 25.00000000000000000 ) ) ;
#2773=AXIS2_PLACEMENT_3D ( 'NONE', #952, #4494, #9812 ) ;
#2807=EDGE_LOOP ( 'NONE', ( #8996, #8842, #8731, #3228, #7372, #7411 ) ) ;
#2808=LINE ( 'NONE', #11646, #7887 ) ;
#2817=CARTESIAN_POINT ( 'NONE',  ( 62.10586122665987574, -20.42344490663940704, -28.00000000000000000 ) ) ;
#2819=ORIENTED_EDGE ( 'NONE', *, *, #7762, .T. ) ;
#2823=ORIENTED_EDGE ( 'NONE', *, *, #10457, .F. ) ;
#2824=CARTESIAN_POINT ( 'NONE',  ( 59.10586122665984732, -20.42344490663941414, 35.00000000000000000 ) ) ;
#2826=ORIENTED_EDGE ( 'NONE', *, *, #3829, .F. ) ;
#2833=FACE_BOUND ( 'NONE', #10951, .T. ) ;
#2838=VERTEX_POINT ( 'NONE', #3561 ) ;
#2842=CIRCLE ( 'NONE', #10995, 2.500000000000002220 ) ;
#2844=DIRECTION ( 'NONE',  ( 1.000000000000000000, 0.000000000000000000, 0.000000000000000000 ) ) ;
#2845=CARTESIAN_POINT ( 'NONE',  ( 54.40514726928103784, 42.68717498692012668, -25.00000000000000000 ) ) ;
#2853=DIRECTION ( 'NONE',  ( 0.000000000000000000, 0.000000000000000000, -1.000000000000000000 ) ) ;
#2860=ORIENTED_EDGE ( 'NONE', *, *, #293, .T. ) ;
#2877=ORIENTED_EDGE ( 'NONE', *, *, #11196, .F. ) ;
#2884=ORIENTED_EDGE ( 'NONE', *, *, #11455, .T. ) ;
#2886=EDGE_LOOP ( 'NONE', ( #9404, #12582, #13083, #11838 ) ) ;
#2898=VERTEX_POINT ( 'NONE', #11435 ) ;
#2902=DIRECTION ( 'NONE',  ( -0.2425356250363330524, 0.9701425001453318764, 0.000000000000000000 ) ) ;
#2903=DIRECTION ( 'NONE',  ( 1.000000000000000000, 0.000000000000000000, 0.000000000000000000 ) ) ;
#2906=CARTESIAN_POINT ( 'NONE',  ( 49.40514726928103073, 42.68717498692012668, 25.00000000000000000 ) ) ;
#2910=AXIS2_PLACEMENT_3D ( 'NONE', #10884, #13237, #10001 ) ;
#2913=FACE_BOUND ( 'NONE', #8983, .T. ) ;
#2914=EDGE_CURVE ( 'NONE', #12288, #10509, #3949, .T. ) ;
#2915=PRODUCT_DEFINITION_FORMATION_WITH_SPECIFIED_SOURCE ( 'ANY', '', #3579, .NOT_KNOWN. ) ;
#2935=ORIENTED_EDGE ( 'NONE', *, *, #5284, .F. ) ;
#2938=ORIENTED_EDGE ( 'NONE', *, *, #3583, .F. ) ;
#2943=DIRECTION ( 'NONE',  ( -0.9701425001453318764, -0.2425356250363329969, 0.000000000000000000 ) ) ;
#2948=DIRECTION ( 'NONE',  ( 1.000000000000000000, 0.000000000000000000, 0.000000000000000000 ) ) ;
#2949=VERTEX_POINT ( 'NONE', #10346 ) ;
#2950=ORIENTED_EDGE ( 'NONE', *, *, #11821, .F. ) ;
#2952=CARTESIAN_POINT ( 'NONE',  ( 59.10586122665984732, -20.42344490663941414, -23.00000000000000000 ) ) ;
#2954=ADVANCED_FACE ( 'NONE', ( #13942 ), #8360, .F. ) ;
#2962=EDGE_LOOP ( 'NONE', ( #5208, #9213, #12484, #4801 ) ) ;
#2965=FACE_OUTER_BOUND ( 'NONE', #7500, .T. ) ;
#2966=DIRECTION ( 'NONE',  ( 0.000000000000000000, -1.000000000000000000, 0.000000000000000000 ) ) ;
#2982=EDGE_CURVE ( 'NONE', #2838, #8043, #2132, .T. ) ;
#3008=EDGE_CURVE ( 'NONE', #3564, #13574, #5345, .T. ) ;
#3012=CIRCLE ( 'NONE', #175, 2.500000000000002220 ) ;
#3025=EDGE_LOOP ( 'NONE', ( #1385, #3637, #7202, #9943 ) ) ;
#3028=ORIENTED_EDGE ( 'NONE', *, *, #3297, .T. ) ;
#3037=DIRECTION ( 'NONE',  ( 0.000000000000000000, 0.000000000000000000, 1.000000000000000000 ) ) ;
#3041=DIRECTION ( 'NONE',  ( 0.000000000000000000, 0.000000000000000000, -1.000000000000000000 ) ) ;
#3048=DIRECTION ( 'NONE',  ( -0.000000000000000000, -0.000000000000000000, -1.000000000000000000 ) ) ;
#3050=VERTEX_POINT ( 'NONE', #3311 ) ;
#3057=ORIENTED_EDGE ( 'NONE', *, *, #9773, .F. ) ;
#3066=DIRECTION ( 'NONE',  ( 0.000000000000000000, 0.000000000000000000, -1.000000000000000000 ) ) ;
#3067=VERTEX_POINT ( 'NONE', #11123 ) ;
#3072=AXIS2_PLACEMENT_3D ( 'NONE', #2513, #1409, #5858 ) ;
#3082=DIRECTION ( 'NONE',  ( 0.2425356250363328026, -0.9701425001453319874, -0.000000000000000000 ) ) ;
#3091=EDGE_CURVE ( 'NONE', #6663, #9400, #11140, .T. ) ;
#3104=VECTOR ( 'NONE', #9548, 1000.000000000000000 ) ;
#3110=VECTOR ( 'NONE', #3603, 1000.000000000000000 ) ;
#3133=CARTESIAN_POINT ( 'NONE',  ( 44.55443476855437268, 62.09002498982675888, 25.00000000000000000 ) ) ;
#3158=ADVANCED_FACE ( 'NONE', ( #12917 ), #13061, .F. ) ;
#3161=ORIENTED_EDGE ( 'NONE', *, *, #356, .T. ) ;
#3167=EDGE_CURVE ( 'NONE', #2838, #1176, #544, .T. ) ;
#3183=FACE_OUTER_BOUND ( 'NONE', #4456, .T. ) ;
#3184=VERTEX_POINT ( 'NONE', #10782 ) ;
#3186=CARTESIAN_POINT ( 'NONE',  ( 39.70372226782770753, 81.49287499273339108, -25.00000000000000000 ) ) ;
#3188=FACE_OUTER_BOUND ( 'NONE', #10770, .T. ) ;
#3189=ORIENTED_EDGE ( 'NONE', *, *, #418, .T. ) ;
#3191=FACE_BOUND ( 'NONE', #14002, .T. ) ;
#3209=FACE_OUTER_BOUND ( 'NONE', #14027, .T. ) ;
#3228=ORIENTED_EDGE ( 'NONE', *, *, #14154, .T. ) ;
#3236=LINE ( 'NONE', #7826, #6818 ) ;
#3243=EDGE_CURVE ( 'NONE', #7740, #12547, #14228, .T. ) ;
#3245=VERTEX_POINT ( 'NONE', #9465 ) ;
#3247=EDGE_CURVE ( 'NONE', #5464, #6880, #7148, .T. ) ;
#3257=SURFACE_SIDE_STYLE ('',( #13363 ) ) ;
#3267=EDGE_CURVE ( 'NONE', #11002, #4176, #11363, .T. ) ;
#3281=ORIENTED_EDGE ( 'NONE', *, *, #3284, .T. ) ;
#3284=EDGE_CURVE ( 'NONE', #4075, #3991, #13253, .T. ) ;
#3297=EDGE_CURVE ( 'NONE', #696, #1781, #12095, .T. ) ;
#3311=CARTESIAN_POINT ( 'NONE',  ( 51.83050351964435976, 32.98574998546678927, -25.00000000000000000 ) ) ;
#3320=VECTOR ( 'NONE', #4898, 1000.000000000000114 ) ;
#3332=ORIENTED_EDGE ( 'NONE', *, *, #2517, .T. ) ;
#3339=STYLED_ITEM ( 'NONE', ( #1054 ), #6268 ) ;
#3341=VECTOR ( 'NONE', #7973, 1000.000000000000000 ) ;
#3350=ADVANCED_FACE ( 'NONE', ( #6442 ), #4357, .T. ) ;
#3357=EDGE_CURVE ( 'NONE', #2898, #4300, #8799, .T. ) ;
#3361=CIRCLE ( 'NONE', #12006, 2.500000000000002220 ) ;
#3362=VERTEX_POINT ( 'NONE', #4435 ) ;
#3376=VECTOR ( 'NONE', #3037, 1000.000000000000000 ) ;
#3388=CARTESIAN_POINT ( 'NONE',  ( 59.18121602037099649, 13.58289998256015352, -25.00000000000000000 ) ) ;
#3398=ORIENTED_EDGE ( 'NONE', *, *, #8557, .F. ) ;
#3401=DIRECTION ( 'NONE',  ( 1.000000000000000000, 0.000000000000000000, 0.000000000000000000 ) ) ;
#3408=ORIENTED_EDGE ( 'NONE', *, *, #3842, .T. ) ;
#3416=CARTESIAN_POINT ( 'NONE',  ( 31.38313257588138683, 143.6985259526510390, 28.00000000000000000 ) ) ;
#3420=VERTEX_POINT ( 'NONE', #13891 ) ;
#3428=VERTEX_POINT ( 'NONE', #271 ) ;
#3431=CARTESIAN_POINT ( 'NONE',  ( 59.10586122665984732, -20.42344490663941414, -35.00000000000000000 ) ) ;
#3441=ADVANCED_FACE ( 'NONE', ( #11529 ), #3714, .F. ) ;
#3450=ORIENTED_EDGE ( 'NONE', *, *, #13375, .F. ) ;
#3460=EDGE_CURVE ( 'NONE', #14384, #12535, #4736, .T. ) ;
#3508=VECTOR ( 'NONE', #6555, 1000.000000000000000 ) ;
#3518=CARTESIAN_POINT ( 'NONE',  ( 71.80728622811317052, -17.99808865627607801, 25.00000000000000000 ) ) ;
#3526=LINE ( 'NONE', #7966, #14072 ) ;
#3553=AXIS2_PLACEMENT_3D ( 'NONE', #13464, #2112, #68 ) ;
#3558=DIRECTION ( 'NONE',  ( 0.000000000000000000, 0.000000000000000000, -1.000000000000000000 ) ) ;
#3560=DIRECTION ( 'NONE',  ( -0.2425356250363327748, 0.9701425001453319874, 0.000000000000000000 ) ) ;
#3561=CARTESIAN_POINT ( 'NONE',  ( 71.80728622811317052, -17.99808865627607801, 25.00000000000000000 ) ) ;
#3564=VERTEX_POINT ( 'NONE', #6459 ) ;
#3579=PRODUCT ( 'Wedge Roller Guide Pins', 'Wedge Roller Guide Pins', '', ( #14066 ) ) ;
#3580=LINE ( 'NONE', #13461, #2750 ) ;
#3583=EDGE_CURVE ( 'NONE', #4300, #2949, #13082, .T. ) ;
#3589=EDGE_LOOP ( 'NONE', ( #5438, #11676, #5797, #921 ) ) ;
#3594=LINE ( 'NONE', #13692, #922 ) ;
#3603=DIRECTION ( 'NONE',  ( -2.243905293393255080E-15, 8.975621173573017164E-15, -1.000000000000000000 ) ) ;
#3608=DIRECTION ( 'NONE',  ( -0.2425356250363327748, 0.9701425001453319874, 0.000000000000000000 ) ) ;
#3613=EDGE_CURVE ( 'NONE', #7164, #4025, #174, .T. ) ;
#3632=ORIENTED_EDGE ( 'NONE', *, *, #9916, .F. ) ;
#3637=ORIENTED_EDGE ( 'NONE', *, *, #4763, .T. ) ;
#3653=LINE ( 'NONE', #4747, #12563 ) ;
#3658=ORIENTED_EDGE ( 'NONE', *, *, #11582, .F. ) ;
#3666=LINE ( 'NONE', #12510, #4702 ) ;
#3670=CARTESIAN_POINT ( 'NONE',  ( 37.35300976710104948, 100.8957249956400375, 25.00000000000000000 ) ) ;
#3680=DIRECTION ( 'NONE',  ( 1.000000000000000000, 0.000000000000000000, 0.000000000000000000 ) ) ;
#3686=EDGE_CURVE ( 'NONE', #3050, #8106, #8460, .T. ) ;
#3694=DIRECTION ( 'NONE',  ( 0.000000000000000000, 1.000000000000000000, 0.000000000000000000 ) ) ;
#3708=VERTEX_POINT ( 'NONE', #2237 ) ;
#3712=ORIENTED_EDGE ( 'NONE', *, *, #5383, .F. ) ;
#3714=PLANE ( 'NONE',  #9634 ) ;
#3715=ORIENTED_EDGE ( 'NONE', *, *, #2397, .T. ) ;
#3729=VERTEX_POINT ( 'NONE', #2302 ) ;
#3733=DIRECTION ( 'NONE',  ( 0.000000000000000000, 0.000000000000000000, 1.000000000000000000 ) ) ;
#3740=ADVANCED_FACE ( 'NONE', ( #10128 ), #114, .T. ) ;
#3744=DIRECTION ( 'NONE',  ( -0.000000000000000000, -0.000000000000000000, -1.000000000000000000 ) ) ;
#3753=CIRCLE ( 'NONE', #14053, 2.500000000000002220 ) ;
#3763=VECTOR ( 'NONE', #3918, 1000.000000000000000 ) ;
#3764=LINE ( 'NONE', #9468, #2460 ) ;
#3775=ORIENTED_EDGE ( 'NONE', *, *, #3091, .F. ) ;
#3777=EDGE_CURVE ( 'NONE', #8106, #3050, #3828, .T. ) ;
#3790=EDGE_LOOP ( 'NONE', ( #3853, #8591 ) ) ;
#3801=CARTESIAN_POINT ( 'NONE',  ( 39.85300976710104948, 100.8957249956400375, -25.00000000000000000 ) ) ;
#3823=PRODUCT_DEFINITION_SHAPE ( 'NONE', 'NONE',  #9731 ) ;
#3824=DIRECTION ( 'NONE',  ( -0.9701425001453319874, -0.2425356250363330801, -0.000000000000000000 ) ) ;
#3826=VERTEX_POINT ( 'NONE', #10408 ) ;
#3828=CIRCLE ( 'NONE', #10116, 2.500000000000002220 ) ;
#3829=EDGE_CURVE ( 'NONE', #5807, #3708, #2737, .T. ) ;
#3830=EDGE_LOOP ( 'NONE', ( #516, #1949 ) ) ;
#3842=EDGE_CURVE ( 'NONE', #3826, #992, #13871, .T. ) ;
#3853=ORIENTED_EDGE ( 'NONE', *, *, #11500, .T. ) ;
#3889=DIRECTION ( 'NONE',  ( 0.000000000000000000, 0.000000000000000000, -1.000000000000000000 ) ) ;
#3894=ORIENTED_EDGE ( 'NONE', *, *, #4568, .F. ) ;
#3900=DIRECTION ( 'NONE',  ( -1.000000000000000000, 0.000000000000000000, 0.000000000000000000 ) ) ;
#3908=DIRECTION ( 'NONE',  ( -1.000000000000000000, 0.000000000000000000, 0.000000000000000000 ) ) ;
#3909=DIRECTION ( 'NONE',  ( 0.000000000000000000, 0.000000000000000000, -1.000000000000000000 ) ) ;
#3918=DIRECTION ( 'NONE',  ( -2.243905293393255080E-15, 8.975621173573017164E-15, -1.000000000000000000 ) ) ;
#3922=ADVANCED_FACE ( 'NONE', ( #2001 ), #4209, .T. ) ;
#3926=DIRECTION ( 'NONE',  ( -0.000000000000000000, -0.000000000000000000, -1.000000000000000000 ) ) ;
#3947=EDGE_CURVE ( 'NONE', #45, #6127, #6164, .T. ) ;
#3949=CIRCLE ( 'NONE', #14000, 2.500000000000002220 ) ;
#3961=CARTESIAN_POINT ( 'NONE',  ( 34.92765351673772045, 110.5971499970933536, 25.00000000000000000 ) ) ;
#3968=DIRECTION ( 'NONE',  ( 0.000000000000000000, 0.000000000000000000, -1.000000000000000000 ) ) ;
#3991=VERTEX_POINT ( 'NONE', #1932 ) ;
#4002=DIRECTION ( 'NONE',  ( 0.000000000000000000, 0.000000000000000000, -1.000000000000000000 ) ) ;
#4016=FACE_OUTER_BOUND ( 'NONE', #12106, .T. ) ;
#4018=CARTESIAN_POINT ( 'NONE',  ( 32.57694101601105530, 130.0000000000000000, -25.00000000000000000 ) ) ;
#4025=VERTEX_POINT ( 'NONE', #1786 ) ;
#4030=ORIENTED_EDGE ( 'NONE', *, *, #11967, .F. ) ;
#4038=FACE_OUTER_BOUND ( 'NONE', #6296, .T. ) ;
#4042=ADVANCED_FACE ( 'NONE', ( #2965 ), #5357, .T. ) ;
#4049=ORIENTED_EDGE ( 'NONE', *, *, #14434, .T. ) ;
#4056=CIRCLE ( 'NONE', #2173, 2.500000000000002220 ) ;
#4057=AXIS2_PLACEMENT_3D ( 'NONE', #1842, #14074, #14147 ) ;
#4075=VERTEX_POINT ( 'NONE', #4574 ) ;
#4078=VERTEX_POINT ( 'NONE', #2224 ) ;
#4090=EDGE_CURVE ( 'NONE', #2107, #4685, #4812, .T. ) ;
#4091=PLANE ( 'NONE',  #9661 ) ;
#4111=ORIENTED_EDGE ( 'NONE', *, *, #10086, .F. ) ;
#4112=DIRECTION ( 'NONE',  ( -0.2425356250363328026, 0.9701425001453319874, 0.000000000000000000 ) ) ;
#4122=VERTEX_POINT ( 'NONE', #4290 ) ;
#4129=CARTESIAN_POINT ( 'NONE',  ( 39.77836601746437850, 91.19429999418670718, -25.00000000000000000 ) ) ;
#4133=DIRECTION ( 'NONE',  ( 0.2425356250363327748, -0.9701425001453319874, -0.000000000000000000 ) ) ;
#4136=DIRECTION ( 'NONE',  ( 0.000000000000000000, 0.000000000000000000, -1.000000000000000000 ) ) ;
#4138=UNCERTAINTY_MEASURE_WITH_UNIT (LENGTH_MEASURE( 1.000000000000000082E-05 ), #5511, 'distance_accuracy_value', 'NONE');
#4174=CARTESIAN_POINT ( 'NONE',  ( 59.10586122665984732, -20.42344490663941414, -35.00000000000000000 ) ) ;
#4176=VERTEX_POINT ( 'NONE', #159 ) ;
#4178=DIRECTION ( 'NONE',  ( -1.000000000000000000, 0.000000000000000000, 0.000000000000000000 ) ) ;
#4179=AXIS2_PLACEMENT_3D ( 'NONE', #5845, #11291, #10184 ) ;
#4181=EDGE_CURVE ( 'NONE', #1781, #3564, #10471, .T. ) ;
#4191=ORIENTED_EDGE ( 'NONE', *, *, #5300, .T. ) ;
#4192=AXIS2_PLACEMENT_3D ( 'NONE', #11228, #1207, #4589 ) ;
#4193=ORIENTED_EDGE ( 'NONE', *, *, #13545, .T. ) ;
#4197=CARTESIAN_POINT ( 'NONE',  ( 31.38313257588138683, 143.6985259526510674, 25.00000000000000000 ) ) ;
#4204=DIRECTION ( 'NONE',  ( -0.9701425001453318764, -0.2425356250363329969, 0.000000000000000000 ) ) ;
#4209=CYLINDRICAL_SURFACE ( 'NONE', #6670, 2.500000000000002220 ) ;
#4211=EDGE_CURVE ( 'NONE', #9931, #2739, #12738, .T. ) ;
#4216=LINE ( 'NONE', #13000, #7509 ) ;
#4221=CARTESIAN_POINT ( 'NONE',  ( 32.50229726637438432, 120.2985749985466839, 25.00000000000000000 ) ) ;
#4230=CARTESIAN_POINT ( 'NONE',  ( 42.27836601746437850, 91.19429999418670718, -25.00000000000000000 ) ) ;
#4241=FACE_OUTER_BOUND ( 'NONE', #1147, .T. ) ;
#4247=ORIENTED_EDGE ( 'NONE', *, *, #75, .T. ) ;
#4250=DIRECTION ( 'NONE',  ( 0.000000000000000000, 0.000000000000000000, -1.000000000000000000 ) ) ;
#4253=ADVANCED_FACE ( 'NONE', ( #7976 ), #2428, .T. ) ;
#4257=AXIS2_PLACEMENT_3D ( 'NONE', #2772, #13964, #12709 ) ;
#4258=CARTESIAN_POINT ( 'NONE',  ( 39.70372226782770753, 81.49287499273339108, 25.00000000000000000 ) ) ;
#4272=ORIENTED_EDGE ( 'NONE', *, *, #4676, .F. ) ;
#4290=CARTESIAN_POINT ( 'NONE',  ( 37.42765351673772045, 110.5971499970933536, -25.00000000000000000 ) ) ;
#4294=DIRECTION ( 'NONE',  ( -1.000000000000000000, 0.000000000000000000, 0.000000000000000000 ) ) ;
#4300=VERTEX_POINT ( 'NONE', #7387 ) ;
#4327=CARTESIAN_POINT ( 'NONE',  ( 62.10586122665984732, -20.42344490663941414, 23.00000000000000000 ) ) ;
#4337=EDGE_CURVE ( 'NONE', #3729, #5373, #11505, .T. ) ;
#4339=EDGE_CURVE ( 'NONE', #908, #55, #10340, .T. ) ;
#4350=DIRECTION ( 'NONE',  ( 0.000000000000000000, -1.000000000000000000, 0.000000000000000000 ) ) ;
#4357=CYLINDRICAL_SURFACE ( 'NONE', #2491, 2.500000000000002220 ) ;
#4365=FILL_AREA_STYLE ('',( #6825 ) ) ;
#4366=EDGE_LOOP ( 'NONE', ( #2297, #9768, #13569, #7829 ) ) ;
#4368=EDGE_CURVE ( 'NONE', #5068, #2603, #812, .T. ) ;
#4379=ADVANCED_FACE ( 'NONE', ( #6221 ), #8335, .F. ) ;
#4386=AXIS2_PLACEMENT_3D ( 'NONE', #1114, #13274, #7545 ) ;
#4391=CARTESIAN_POINT ( 'NONE',  ( 62.10586122665987574, -20.42344490663940704, 28.00000000000000000 ) ) ;
#4398=DIRECTION ( 'NONE',  ( 0.000000000000000000, 0.000000000000000000, -1.000000000000000000 ) ) ;
#4400=CYLINDRICAL_SURFACE ( 'NONE', #1439, 2.500000000000002220 ) ;
#4422=LINE ( 'NONE', #8852, #3320 ) ;
#4423=EDGE_LOOP ( 'NONE', ( #11808, #3715, #558, #1090, #12995, #12520 ) ) ;
#4435=CARTESIAN_POINT ( 'NONE',  ( 42.12907851819100813, 71.79144999128007498, 25.00000000000000000 ) ) ;
#4440=ORIENTED_EDGE ( 'NONE', *, *, #6384, .F. ) ;
#4443=ORIENTED_EDGE ( 'NONE', *, *, #3460, .F. ) ;
#4456=EDGE_LOOP ( 'NONE', ( #11312, #11868, #10925, #11480 ) ) ;
#4458=CARTESIAN_POINT ( 'NONE',  ( 21.68170757442808849, 141.2731697022877313, 28.00000000000000000 ) ) ;
#4459=AXIS2_PLACEMENT_3D ( 'NONE', #1095, #4485, #8919 ) ;
#4466=VERTEX_POINT ( 'NONE', #9803 ) ;
#4469=CYLINDRICAL_SURFACE ( 'NONE', #10965, 2.500000000000002220 ) ;
#4474=DIRECTION ( 'NONE',  ( 1.000000000000000000, 0.000000000000000000, 0.000000000000000000 ) ) ;
#4475=AXIS2_PLACEMENT_3D ( 'NONE', #5801, #2539, #12775 ) ;
#4479=DIRECTION ( 'NONE',  ( -0.2425356250363327748, 0.9701425001453319874, 0.000000000000000000 ) ) ;
#4480=CIRCLE ( 'NONE', #11947, 2.500000000000009326 ) ;
#4485=DIRECTION ( 'NONE',  ( 0.000000000000000000, 0.000000000000000000, -1.000000000000000000 ) ) ;
#4494=DIRECTION ( 'NONE',  ( 0.000000000000000000, 0.000000000000000000, -1.000000000000000000 ) ) ;
#4518=VERTEX_POINT ( 'NONE', #1094 ) ;
#4519=CARTESIAN_POINT ( 'NONE',  ( 47.12907851819101523, 71.79144999128007498, -25.00000000000000000 ) ) ;
#4535=AXIS2_PLACEMENT_3D ( 'NONE', #12310, #10981, #956 ) ;
#4546=CARTESIAN_POINT ( 'NONE',  ( 64.03192852109765454, -5.819950020346492892, 25.00000000000000000 ) ) ;
#4555=ORIENTED_EDGE ( 'NONE', *, *, #4763, .F. ) ;
#4568=EDGE_CURVE ( 'NONE', #1702, #12288, #12015, .T. ) ;
#4574=CARTESIAN_POINT ( 'NONE',  ( 59.25585977000769589, 23.28432498401347672, 25.00000000000000000 ) ) ;
#4585=CARTESIAN_POINT ( 'NONE',  ( 59.18121602037099649, 13.58289998256015352, 25.00000000000000000 ) ) ;
#4589=DIRECTION ( 'NONE',  ( -1.000000000000000000, 0.000000000000000000, 0.000000000000000000 ) ) ;
#4593=LINE ( 'NONE', #8002, #8820 ) ;
#4600=EDGE_CURVE ( 'NONE', #4518, #1328, #13764, .T. ) ;
#4601=EDGE_LOOP ( 'NONE', ( #10210, #5875, #830, #7535 ) ) ;
#4606=CARTESIAN_POINT ( 'NONE',  ( 42.20372226782770753, 81.49287499273339108, 25.00000000000000000 ) ) ;
#4616=FACE_OUTER_BOUND ( 'NONE', #5685, .T. ) ;
#4627=PLANE ( 'NONE',  #13165 ) ;
#4636=AXIS2_PLACEMENT_3D ( 'NONE', #7038, #13876, #10415 ) ;
#4643=EDGE_LOOP ( 'NONE', ( #12354, #6102, #5914, #12049 ) ) ;
#4663=EDGE_CURVE ( 'NONE', #4769, #55, #12642, .T. ) ;
#4676=EDGE_CURVE ( 'NONE', #1176, #12547, #2633, .T. ) ;
#4677=EDGE_CURVE ( 'NONE', #12519, #10509, #12570, .T. ) ;
#4685=VERTEX_POINT ( 'NONE', #10447 ) ;
#4702=VECTOR ( 'NONE', #7007, 1000.000000000000000 ) ;
#4716=DIRECTION ( 'NONE',  ( -1.000000000000000000, 0.000000000000000000, 0.000000000000000000 ) ) ;
#4717=PLANE ( 'NONE',  #3072 ) ;
#4724=EDGE_LOOP ( 'NONE', ( #10248, #3408, #10323, #7341 ) ) ;
#4726=AXIS2_PLACEMENT_3D ( 'NONE', #6179, #10651, #8445 ) ;
#4729=ADVANCED_FACE ( 'NONE', ( #4616 ), #9057, .T. ) ;
#4736=LINE ( 'NONE', #12701, #10795 ) ;
#4746=DIRECTION ( 'NONE',  ( -1.000000000000000000, 0.000000000000000000, 0.000000000000000000 ) ) ;
#4747=CARTESIAN_POINT ( 'NONE',  ( 37.42765351673772045, 110.5971499970933536, 25.00000000000000000 ) ) ;
#4754=DIRECTION ( 'NONE',  ( 0.000000000000000000, 0.000000000000000000, -1.000000000000000000 ) ) ;
#4763=EDGE_CURVE ( 'NONE', #6682, #8106, #1679, .T. ) ;
#4765=LINE ( 'NONE', #2720, #3110 ) ;
#4769=VERTEX_POINT ( 'NONE', #12051 ) ;
#4801=ORIENTED_EDGE ( 'NONE', *, *, #2205, .T. ) ;
#4812=CIRCLE ( 'NONE', #8552, 2.500000000000002220 ) ;
#4821=CARTESIAN_POINT ( 'NONE',  ( 30.07694101601105530, 130.0000000000000000, 25.00000000000000000 ) ) ;
#4828=DIRECTION ( 'NONE',  ( 1.000000000000000000, 0.000000000000000000, 0.000000000000000000 ) ) ;
#4835=CARTESIAN_POINT ( 'NONE',  ( 37.35300976710104948, 100.8957249956400375, 25.00000000000000000 ) ) ;
#4836=FACE_OUTER_BOUND ( 'NONE', #2007, .T. ) ;
#4840=CIRCLE ( 'NONE', #10693, 2.500000000000009326 ) ;
#4849=CARTESIAN_POINT ( 'NONE',  ( 51.97979101891770171, 52.38859998837343568, 25.00000000000000000 ) ) ;
#4853=DIRECTION ( 'NONE',  ( 0.9701425001453318764, 0.2425356250363329969, 0.000000000000000000 ) ) ;
#4876=DIRECTION ( 'NONE',  ( -1.000000000000000000, 0.000000000000000000, 0.000000000000000000 ) ) ;
#4877=CYLINDRICAL_SURFACE ( 'NONE', #1595, 2.500000000000002220 ) ;
#4881=CARTESIAN_POINT ( 'NONE',  ( 62.10586122665987574, -20.42344490663940704, 28.00000000000000000 ) ) ;
#4886=VECTOR ( 'NONE', #7078, 1000.000000000000114 ) ;
#4892=DIRECTION ( 'NONE',  ( 0.000000000000000000, 0.000000000000000000, -1.000000000000000000 ) ) ;
#4895=LINE ( 'NONE', #8254, #11957 ) ;
#4898=DIRECTION ( 'NONE',  ( -0.9701425001453318764, -0.2425356250363329969, 0.000000000000000000 ) ) ;
#4900=EDGE_CURVE ( 'NONE', #7164, #3184, #13997, .T. ) ;
#4902=FACE_OUTER_BOUND ( 'NONE', #11077, .T. ) ;
#4914=AXIS2_PLACEMENT_3D ( 'NONE', #4606, #7947, #2695 ) ;
#4915=DIRECTION ( 'NONE',  ( -0.9701425001453319874, -0.2425356250363330801, 0.000000000000000000 ) ) ;
#4933=ORIENTED_EDGE ( 'NONE', *, *, #2729, .T. ) ;
#4971=EDGE_CURVE ( 'NONE', #5200, #2033, #7852, .T. ) ;
#4982=ORIENTED_EDGE ( 'NONE', *, *, #13259, .F. ) ;
#5000=CARTESIAN_POINT ( 'NONE',  ( 62.10586122665984732, -20.42344490663941414, -23.00000000000000000 ) ) ;
#5010=CARTESIAN_POINT ( 'NONE',  ( 59.10586122665984732, -20.42344490663941414, -23.00000000000000000 ) ) ;
#5017=EDGE_LOOP ( 'NONE', ( #10657, #2045, #12635, #9101 ) ) ;
#5019=FACE_BOUND ( 'NONE', #3790, .T. ) ;
#5032=LINE ( 'NONE', #13827, #6791 ) ;
#5043=DIRECTION ( 'NONE',  ( 0.000000000000000000, 0.000000000000000000, -1.000000000000000000 ) ) ;
#5052=ADVANCED_FACE ( 'NONE', ( #11433 ), #7261, .T. ) ;
#5067=CARTESIAN_POINT ( 'NONE',  ( 71.80728622811317052, -17.99808865627607801, 25.00000000000000000 ) ) ;
#5068=VERTEX_POINT ( 'NONE', #5010 ) ;
#5070=CARTESIAN_POINT ( 'NONE',  ( 62.10586122665984732, -20.42344490663941414, -35.00000000000000000 ) ) ;
#5080=EDGE_CURVE ( 'NONE', #12535, #3564, #3764, .T. ) ;
#5081=FACE_BOUND ( 'NONE', #6073, .T. ) ;
#5087=ORIENTED_EDGE ( 'NONE', *, *, #3091, .T. ) ;
#5119=CARTESIAN_POINT ( 'NONE',  ( 18.68170757442808849, 141.2731697022877313, -35.00000000000000000 ) ) ;
#5121=ORIENTED_EDGE ( 'NONE', *, *, #7478, .F. ) ;
#5123=ORIENTED_EDGE ( 'NONE', *, *, #1819, .T. ) ;
#5124=ORIENTED_EDGE ( 'NONE', *, *, #9852, .T. ) ;
#5131=AXIS2_PLACEMENT_3D ( 'NONE', #10472, #453, #10548 ) ;
#5134=LINE ( 'NONE', #7327, #9301 ) ;
#5161=CARTESIAN_POINT ( 'NONE',  ( 71.80728622811317052, -17.99808865627607801, 25.00000000000000000 ) ) ;
#5196=CIRCLE ( 'NONE', #14089, 2.500000000000002220 ) ;
#5200=VERTEX_POINT ( 'NONE', #5070 ) ;
#5201=DIRECTION ( 'NONE',  ( -1.000000000000000000, 0.000000000000000000, 0.000000000000000000 ) ) ;
#5206=EDGE_CURVE ( 'NONE', #4122, #10954, #884, .T. ) ;
#5208=ORIENTED_EDGE ( 'NONE', *, *, #4181, .T. ) ;
#5212=DIRECTION ( 'NONE',  ( -1.000000000000000000, 0.000000000000000000, 0.000000000000000000 ) ) ;
#5217=CARTESIAN_POINT ( 'NONE',  ( 62.10586122665984732, -20.42344490663941414, 25.00000000000000000 ) ) ;
#5258=LINE ( 'NONE', #4391, #13431 ) ;
#5262=LINE ( 'NONE', #4327, #3508 ) ;
#5275=ORIENTED_EDGE ( 'NONE', *, *, #8646, .T. ) ;
#5282=LINE ( 'NONE', #5352, #5640 ) ;
#5284=EDGE_CURVE ( 'NONE', #5967, #7049, #3594, .T. ) ;
#5298=DIRECTION ( 'NONE',  ( -0.2425356250363330801, 0.9701425001453319874, 0.000000000000000000 ) ) ;
#5300=EDGE_CURVE ( 'NONE', #1210, #992, #12382, .T. ) ;
#5345=LINE ( 'NONE', #2211, #10438 ) ;
#5351=FACE_OUTER_BOUND ( 'NONE', #12690, .T. ) ;
#5352=CARTESIAN_POINT ( 'NONE',  ( 62.10586122665984732, -20.42344490663941414, 23.00000000000000000 ) ) ;
#5357=PLANE ( 'NONE',  #1813 ) ;
#5371=FACE_BOUND ( 'NONE', #6212, .T. ) ;
#5373=VERTEX_POINT ( 'NONE', #591 ) ;
#5379=DIRECTION ( 'NONE',  ( 0.000000000000000000, 0.000000000000000000, -1.000000000000000000 ) ) ;
#5383=EDGE_CURVE ( 'NONE', #12126, #260, #1676, .T. ) ;
#5397=DIRECTION ( 'NONE',  ( -2.243905293393255080E-15, 8.975621173573017164E-15, 1.000000000000000000 ) ) ;
#5405=AXIS2_PLACEMENT_3D ( 'NONE', #8193, #11490, #12584 ) ;
#5411=AXIS2_PLACEMENT_3D ( 'NONE', #9660, #6283, #7383 ) ;
#5422=FACE_OUTER_BOUND ( 'NONE', #11714, .T. ) ;
#5438=ORIENTED_EDGE ( 'NONE', *, *, #674, .T. ) ;
#5440=VECTOR ( 'NONE', #7656, 1000.000000000000000 ) ;
#5441=DIRECTION ( 'NONE',  ( 1.000000000000000000, 0.000000000000000000, 0.000000000000000000 ) ) ;
#5442=ORIENTED_EDGE ( 'NONE', *, *, #11403, .F. ) ;
#5444=CARTESIAN_POINT ( 'NONE',  ( 51.83050351964435976, 32.98574998546678927, 25.00000000000000000 ) ) ;
#5445=ORIENTED_EDGE ( 'NONE', *, *, #12914, .F. ) ;
#5446=ORIENTED_EDGE ( 'NONE', *, *, #1453, .F. ) ;
#5464=VERTEX_POINT ( 'NONE', #6276 ) ;
#5475=CARTESIAN_POINT ( 'NONE',  ( 34.92765351673772045, 110.5971499970933536, 25.00000000000000000 ) ) ;
#5476=VECTOR ( 'NONE', #4479, 999.9999999999998863 ) ;
#5511=( LENGTH_UNIT ( ) NAMED_UNIT ( * ) SI_UNIT ( .MILLI., .METRE. ) );
#5519=DIRECTION ( 'NONE',  ( -1.000000000000000000, 0.000000000000000000, 0.000000000000000000 ) ) ;
#5523=DIRECTION ( 'NONE',  ( 0.000000000000000000, 0.000000000000000000, -1.000000000000000000 ) ) ;
#5535=DIRECTION ( 'NONE',  ( -1.000000000000000000, 0.000000000000000000, 0.000000000000000000 ) ) ;
#5544=ORIENTED_EDGE ( 'NONE', *, *, #1198, .F. ) ;
#5546=CARTESIAN_POINT ( 'NONE',  ( 37.27836601746437850, 91.19429999418670718, -25.00000000000000000 ) ) ;
#5556=DIRECTION ( 'NONE',  ( -1.000000000000000000, 0.000000000000000000, 0.000000000000000000 ) ) ;
#5566=CYLINDRICAL_SURFACE ( 'NONE', #2355, 2.500000000000002220 ) ;
#5567=DIRECTION ( 'NONE',  ( -1.000000000000000000, 0.000000000000000000, 0.000000000000000000 ) ) ;
#5578=CARTESIAN_POINT ( 'NONE',  ( 49.47979101891770171, 52.38859998837343568, -25.00000000000000000 ) ) ;
#5607=DIRECTION ( 'NONE',  ( 0.000000000000000000, 0.000000000000000000, 1.000000000000000000 ) ) ;
#5618=VERTEX_POINT ( 'NONE', #11170 ) ;
#5638=DIRECTION ( 'NONE',  ( -1.000000000000000000, 0.000000000000000000, 0.000000000000000000 ) ) ;
#5640=VECTOR ( 'NONE', #6226, 1000.000000000000000 ) ;
#5645=EDGE_CURVE ( 'NONE', #4075, #2107, #12130, .T. ) ;
#5673=CIRCLE ( 'NONE', #13881, 2.500000000000002220 ) ;
#5685=EDGE_LOOP ( 'NONE', ( #4272, #14100, #13025, #8572 ) ) ;
#5701=DIRECTION ( 'NONE',  ( -1.000000000000000000, 0.000000000000000000, 0.000000000000000000 ) ) ;
#5704=ORIENTED_EDGE ( 'NONE', *, *, #10484, .F. ) ;
#5720=EDGE_LOOP ( 'NONE', ( #12901, #7725, #3398, #14421 ) ) ;
#5721=CYLINDRICAL_SURFACE ( 'NONE', #7165, 2.500000000000002220 ) ;
#5722=EDGE_CURVE ( 'NONE', #192, #13539, #8645, .T. ) ;
#5741=ORIENTED_EDGE ( 'NONE', *, *, #8752, .T. ) ;
#5754=ORIENTED_EDGE ( 'NONE', *, *, #8528, .F. ) ;
#5764=ORIENTED_EDGE ( 'NONE', *, *, #1851, .T. ) ;
#5765=ORIENTED_EDGE ( 'NONE', *, *, #13086, .F. ) ;
#5769=EDGE_CURVE ( 'NONE', #3428, #1985, #10765, .T. ) ;
#5784=FACE_OUTER_BOUND ( 'NONE', #9759, .T. ) ;
#5788=LINE ( 'NONE', #13803, #12630 ) ;
#5789=ORIENTED_EDGE ( 'NONE', *, *, #13199, .F. ) ;
#5797=ORIENTED_EDGE ( 'NONE', *, *, #2348, .T. ) ;
#5801=CARTESIAN_POINT ( 'NONE',  ( 32.50229726637438432, 120.2985749985466839, 25.00000000000000000 ) ) ;
#5807=VERTEX_POINT ( 'NONE', #13744 ) ;
#5808=CARTESIAN_POINT ( 'NONE',  ( 47.05443476855437268, 62.09002498982675888, -25.00000000000000000 ) ) ;
#5810=DIRECTION ( 'NONE',  ( -0.000000000000000000, -0.000000000000000000, -1.000000000000000000 ) ) ;
#5826=CYLINDRICAL_SURFACE ( 'NONE', #8197, 2.500000000000002220 ) ;
#5843=AXIS2_PLACEMENT_3D ( 'NONE', #10757, #14139, #10894 ) ;
#5844=ORIENTED_EDGE ( 'NONE', *, *, #7715, .T. ) ;
#5845=CARTESIAN_POINT ( 'NONE',  ( 34.92765351673772045, 110.5971499970933536, 25.00000000000000000 ) ) ;
#5848=ORIENTED_EDGE ( 'NONE', *, *, #3777, .F. ) ;
#5858=DIRECTION ( 'NONE',  ( -1.000000000000000000, 0.000000000000000000, 0.000000000000000000 ) ) ;
#5865=CARTESIAN_POINT ( 'NONE',  ( 44.70372226782771463, 81.49287499273339108, 25.00000000000000000 ) ) ;
#5866=AXIS2_PLACEMENT_3D ( 'NONE', #461, #4915, #9379 ) ;
#5874=ORIENTED_EDGE ( 'NONE', *, *, #12278, .F. ) ;
#5875=ORIENTED_EDGE ( 'NONE', *, *, #12402, .T. ) ;
#5882=DIRECTION ( 'NONE',  ( 0.000000000000000000, 0.000000000000000000, -1.000000000000000000 ) ) ;
#5884=AXIS2_PLACEMENT_3D ( 'NONE', #6366, #3968, #7454 ) ;
#5887=CARTESIAN_POINT ( 'NONE',  ( 21.68170757442808849, 141.2731697022877313, -23.00000000000000000 ) ) ;
#5891=DIRECTION ( 'NONE',  ( 0.000000000000000000, 0.000000000000000000, -1.000000000000000000 ) ) ;
#5901=CARTESIAN_POINT ( 'NONE',  ( 39.85300976710104948, 100.8957249956400375, 25.00000000000000000 ) ) ;
#5914=ORIENTED_EDGE ( 'NONE', *, *, #1266, .F. ) ;
#5917=ORIENTED_EDGE ( 'NONE', *, *, #4090, .T. ) ;
#5939=EDGE_LOOP ( 'NONE', ( #9272, #4933, #971, #5442 ) ) ;
#5944=ORIENTED_EDGE ( 'NONE', *, *, #10036, .F. ) ;
#5946=PLANE ( 'NONE',  #12231 ) ;
#5967=VERTEX_POINT ( 'NONE', #3416 ) ;
#5987=AXIS2_PLACEMENT_3D ( 'NONE', #2693, #13960, #4876 ) ;
#6011=CARTESIAN_POINT ( 'NONE',  ( 21.68170757442806362, 141.2731697022877029, 28.00000000000000000 ) ) ;
#6012=EDGE_LOOP ( 'NONE', ( #5544, #9835, #13604, #3775 ) ) ;
#6020=ORIENTED_EDGE ( 'NONE', *, *, #11046, .F. ) ;
#6022=CARTESIAN_POINT ( 'NONE',  ( 30.07694101601105530, 130.0000000000000000, 25.00000000000000000 ) ) ;
#6028=ORIENTED_EDGE ( 'NONE', *, *, #10036, .T. ) ;
#6040=CARTESIAN_POINT ( 'NONE',  ( 56.83050351964436686, 32.98574998546678927, -25.00000000000000000 ) ) ;
#6048=DIRECTION ( 'NONE',  ( 0.2425356250363327748, -0.9701425001453319874, -0.000000000000000000 ) ) ;
#6073=EDGE_LOOP ( 'NONE', ( #10862, #5087 ) ) ;
#6081=( GEOMETRIC_REPRESENTATION_CONTEXT ( 3 ) GLOBAL_UNCERTAINTY_ASSIGNED_CONTEXT ( ( #13656 ) ) GLOBAL_UNIT_ASSIGNED_CONTEXT ( ( #13449, #6542, #7635 ) ) REPRESENTATION_CONTEXT ( 'NONE', 'WORKASPACE' ) );
#6095=AXIS2_PLACEMENT_3D ( 'NONE', #217, #10388, #10534 ) ;
#6102=ORIENTED_EDGE ( 'NONE', *, *, #1198, .T. ) ;
#6114=PLANE ( 'NONE',  #1587 ) ;
#6119=ADVANCED_FACE ( 'NONE', ( #5784 ), #4717, .T. ) ;
#6127=VERTEX_POINT ( 'NONE', #1935 ) ;
#6131=DIRECTION ( 'NONE',  ( 0.000000000000000000, 0.000000000000000000, -1.000000000000000000 ) ) ;
#6164=LINE ( 'NONE', #2817, #13011 ) ;
#6171=LINE ( 'NONE', #10646, #3104 ) ;
#6179=CARTESIAN_POINT ( 'NONE',  ( 21.68170757442808849, 141.2731697022877313, 23.00000000000000000 ) ) ;
#6183=FACE_BOUND ( 'NONE', #9597, .T. ) ;
#6185=DIRECTION ( 'NONE',  ( 1.000000000000000000, 0.000000000000000000, 0.000000000000000000 ) ) ;
#6189=EDGE_CURVE ( 'NONE', #2033, #6127, #12753, .T. ) ;
#6194=DIRECTION ( 'NONE',  ( -1.000000000000000000, 0.000000000000000000, 0.000000000000000000 ) ) ;
#6212=EDGE_LOOP ( 'NONE', ( #10073, #9171 ) ) ;
#6221=FACE_OUTER_BOUND ( 'NONE', #4366, .T. ) ;
#6226=DIRECTION ( 'NONE',  ( 0.000000000000000000, 0.000000000000000000, 1.000000000000000000 ) ) ;
#6252=ORIENTED_EDGE ( 'NONE', *, *, #11582, .T. ) ;
#6259=CYLINDRICAL_SURFACE ( 'NONE', #5987, 2.500000000000002220 ) ;
#6265=CIRCLE ( 'NONE', #13532, 2.500000000000002220 ) ;
#6267=CIRCLE ( 'NONE', #1351, 2.500000000000002220 ) ;
#6268=ADVANCED_BREP_SHAPE_REPRESENTATION ( '', ( #11686, #11025 ), #12660 ) ;
#6276=CARTESIAN_POINT ( 'NONE',  ( 49.40514726928103073, 42.68717498692012668, -25.00000000000000000 ) ) ;
#6278=FACE_OUTER_BOUND ( 'NONE', #13428, .T. ) ;
#6283=DIRECTION ( 'NONE',  ( 0.000000000000000000, 0.000000000000000000, -1.000000000000000000 ) ) ;
#6296=EDGE_LOOP ( 'NONE', ( #11156, #5741, #6787, #5765 ) ) ;
#6299=CARTESIAN_POINT ( 'NONE',  ( 64.03192852109765454, -5.819950020346492892, 25.00000000000000000 ) ) ;
#6308=CARTESIAN_POINT ( 'NONE',  ( 18.68170757442808849, 141.2731697022877313, -35.00000000000000000 ) ) ;
#6366=CARTESIAN_POINT ( 'NONE',  ( 32.50229726637438432, 120.2985749985466839, -25.00000000000000000 ) ) ;
#6375=DIRECTION ( 'NONE',  ( -1.000000000000000000, 0.000000000000000000, 0.000000000000000000 ) ) ;
#6384=EDGE_CURVE ( 'NONE', #8545, #2739, #8176, .T. ) ;
#6401=ADVANCED_FACE ( 'NONE', ( #6817 ), #11697, .T. ) ;
#6411=CARTESIAN_POINT ( 'NONE',  ( 32.50229726637438432, 120.2985749985466839, 25.00000000000000000 ) ) ;
#6418=CARTESIAN_POINT ( 'NONE',  ( 49.47979101891770171, 52.38859998837343568, 25.00000000000000000 ) ) ;
#6424=CARTESIAN_POINT ( 'NONE',  ( 34.85300976710104948, 100.8957249956400375, -25.00000000000000000 ) ) ;
#6427=CARTESIAN_POINT ( 'NONE',  ( 62.10586122665984732, -20.42344490663941414, 35.00000000000000000 ) ) ;
#6433=DIRECTION ( 'NONE',  ( 0.000000000000000000, 0.000000000000000000, -1.000000000000000000 ) ) ;
#6436=LINE ( 'NONE', #8644, #3376 ) ;
#6442=FACE_OUTER_BOUND ( 'NONE', #12476, .T. ) ;
#6457=ORIENTED_EDGE ( 'NONE', *, *, #12716, .F. ) ;
#6459=CARTESIAN_POINT ( 'NONE',  ( 18.68170757442808849, 141.2731697022877313, 23.00000000000000000 ) ) ;
#6468=ORIENTED_EDGE ( 'NONE', *, *, #9520, .T. ) ;
#6469=CARTESIAN_POINT ( 'NONE',  ( 49.55443476855437268, 62.09002498982675888, -25.00000000000000000 ) ) ;
#6472=EDGE_CURVE ( 'NONE', #3067, #45, #8253, .T. ) ;
#6477=DIRECTION ( 'NONE',  ( 0.9701425001453319874, 0.2425356250363328026, 0.000000000000000000 ) ) ;
#6485=CARTESIAN_POINT ( 'NONE',  ( 71.80728622811317052, -17.99808865627607801, 28.00000000000000000 ) ) ;
#6514=DIRECTION ( 'NONE',  ( -1.000000000000000000, 0.000000000000000000, 0.000000000000000000 ) ) ;
#6516=CARTESIAN_POINT ( 'NONE',  ( 59.18121602037099649, 13.58289998256015352, 25.00000000000000000 ) ) ;
#6524=DIRECTION ( 'NONE',  ( 0.000000000000000000, 0.000000000000000000, 1.000000000000000000 ) ) ;
#6525=VECTOR ( 'NONE', #2108, 1000.000000000000000 ) ;
#6528=DIRECTION ( 'NONE',  ( -1.000000000000000000, 0.000000000000000000, 0.000000000000000000 ) ) ;
#6542=( NAMED_UNIT ( * ) PLANE_ANGLE_UNIT ( ) SI_UNIT ( $, .RADIAN. ) );
#6555=DIRECTION ( 'NONE',  ( -1.000000000000000000, 0.000000000000000000, 0.000000000000000000 ) ) ;
#6557=ADVANCED_FACE ( 'NONE', ( #6278 ), #10751, .F. ) ;
#6568=ORIENTED_EDGE ( 'NONE', *, *, #12402, .F. ) ;
#6575=LINE ( 'NONE', #4197, #13326 ) ;
#6595=DIRECTION ( 'NONE',  ( -0.000000000000000000, -0.000000000000000000, -1.000000000000000000 ) ) ;
#6610=CARTESIAN_POINT ( 'NONE',  ( 54.33050351964436686, 32.98574998546678927, -25.00000000000000000 ) ) ;
#6625=ORIENTED_EDGE ( 'NONE', *, *, #4663, .T. ) ;
#6640=FACE_OUTER_BOUND ( 'NONE', #11690, .T. ) ;
#6651=CYLINDRICAL_SURFACE ( 'NONE', #4459, 2.500000000000002220 ) ;
#6660=CYLINDRICAL_SURFACE ( 'NONE', #13857, 2.500000000000002220 ) ;
#6663=VERTEX_POINT ( 'NONE', #2110 ) ;
#6664=DIRECTION ( 'NONE',  ( -1.000000000000000000, 0.000000000000000000, 0.000000000000000000 ) ) ;
#6665=DIRECTION ( 'NONE',  ( 0.000000000000000000, 0.000000000000000000, -1.000000000000000000 ) ) ;
#6666=CARTESIAN_POINT ( 'NONE',  ( 56.75585977000769589, 23.28432498401347672, 25.00000000000000000 ) ) ;
#6667=ADVANCED_FACE ( 'NONE', ( #2191 ), #4469, .T. ) ;
#6670=AXIS2_PLACEMENT_3D ( 'NONE', #11954, #13060, #3908 ) ;
#6676=( NAMED_UNIT ( * ) PLANE_ANGLE_UNIT ( ) SI_UNIT ( $, .RADIAN. ) );
#6680=ORIENTED_EDGE ( 'NONE', *, *, #6989, .T. ) ;
#6682=VERTEX_POINT ( 'NONE', #9937 ) ;
#6683=ORIENTED_EDGE ( 'NONE', *, *, #6831, .F. ) ;
#6688=CARTESIAN_POINT ( 'NONE',  ( 21.68170757442806362, 141.2731697022877313, -25.00000000000000000 ) ) ;
#6703=DIRECTION ( 'NONE',  ( -0.9701425001453319874, -0.2425356250363327471, 0.000000000000000000 ) ) ;
#6709=DIRECTION ( 'NONE',  ( -0.000000000000000000, -0.000000000000000000, -1.000000000000000000 ) ) ;
#6712=ADVANCED_FACE ( 'NONE', ( #10006 ), #14410, .T. ) ;
#6713=ORIENTED_EDGE ( 'NONE', *, *, #12716, .T. ) ;
#6724=CARTESIAN_POINT ( 'NONE',  ( 71.80728622811317052, -17.99808865627607801, 25.00000000000000000 ) ) ;
#6730=EDGE_LOOP ( 'NONE', ( #12509, #1221 ) ) ;
#6744=ADVANCED_FACE ( 'NONE', ( #2259 ), #12351, .F. ) ;
#6747=DIRECTION ( 'NONE',  ( -2.243905293393255080E-15, 8.975621173573017164E-15, 1.000000000000000000 ) ) ;
#6750=ORIENTED_EDGE ( 'NONE', *, *, #4339, .F. ) ;
#6763=LINE ( 'NONE', #7636, #7912 ) ;
#6785=AXIS2_PLACEMENT_3D ( 'NONE', #8857, #4002, #6664 ) ;
#6786=FACE_BOUND ( 'NONE', #7453, .T. ) ;
#6787=ORIENTED_EDGE ( 'NONE', *, *, #14125, .F. ) ;
#6791=VECTOR ( 'NONE', #11769, 1000.000000000000000 ) ;
#6816=VECTOR ( 'NONE', #8744, 1000.000000000000000 ) ;
#6817=FACE_OUTER_BOUND ( 'NONE', #13441, .T. ) ;
#6818=VECTOR ( 'NONE', #13418, 1000.000000000000000 ) ;
#6825=FILL_AREA_STYLE_COLOUR ( '', #11491 ) ;
#6828=VECTOR ( 'NONE', #13116, 1000.000000000000000 ) ;
#6831=EDGE_CURVE ( 'NONE', #5807, #11937, #8841, .T. ) ;
#6851=ORIENTED_EDGE ( 'NONE', *, *, #12017, .T. ) ;
#6872=DIRECTION ( 'NONE',  ( 0.2425356250363329969, -0.9701425001453318764, -0.000000000000000000 ) ) ;
#6879=DIRECTION ( 'NONE',  ( -0.9701425001453318764, -0.2425356250363329969, 0.000000000000000000 ) ) ;
#6880=VERTEX_POINT ( 'NONE', #2845 ) ;
#6888=EDGE_LOOP ( 'NONE', ( #4191, #7370 ) ) ;
#6893=EDGE_LOOP ( 'NONE', ( #2823, #5754 ) ) ;
#6924=AXIS2_PLACEMENT_3D ( 'NONE', #6666, #11205, #10986 ) ;
#6946=CIRCLE ( 'NONE', #666, 2.500000000000002220 ) ;
#6953=EDGE_LOOP ( 'NONE', ( #5446, #10052, #10764, #13861 ) ) ;
#6956=ORIENTED_EDGE ( 'NONE', *, *, #9916, .T. ) ;
#6961=CARTESIAN_POINT ( 'NONE',  ( 54.33050351964436686, 32.98574998546678927, -25.00000000000000000 ) ) ;
#6966=ORIENTED_EDGE ( 'NONE', *, *, #8646, .F. ) ;
#6988=DIRECTION ( 'NONE',  ( 0.000000000000000000, 0.000000000000000000, -1.000000000000000000 ) ) ;
#6989=EDGE_CURVE ( 'NONE', #696, #7740, #6763, .T. ) ;
#7005=VECTOR ( 'NONE', #5607, 1000.000000000000000 ) ;
#7007=DIRECTION ( 'NONE',  ( 0.000000000000000000, 0.000000000000000000, -1.000000000000000000 ) ) ;
#7018=CARTESIAN_POINT ( 'NONE',  ( 31.38313257588138683, 143.6985259526510674, -25.00000000000000000 ) ) ;
#7026=FACE_OUTER_BOUND ( 'NONE', #5720, .T. ) ;
#7038=CARTESIAN_POINT ( 'NONE',  ( 49.47979101891770171, 52.38859998837343568, 25.00000000000000000 ) ) ;
#7049=VERTEX_POINT ( 'NONE', #4458 ) ;
#7058=VECTOR ( 'NONE', #2163, 1000.000000000000000 ) ;
#7065=CARTESIAN_POINT ( 'NONE',  ( 18.68170757442808849, 141.2731697022877313, 35.00000000000000000 ) ) ;
#7078=DIRECTION ( 'NONE',  ( -0.9701425001453318764, -0.2425356250363329969, 0.000000000000000000 ) ) ;
#7079=CARTESIAN_POINT ( 'NONE',  ( 31.38313257588138683, 143.6985259526510390, -28.00000000000000000 ) ) ;
#7083=CARTESIAN_POINT ( 'NONE',  ( 54.33050351964436686, 32.98574998546678927, 25.00000000000000000 ) ) ;
#7084=CIRCLE ( 'NONE', #2910, 2.500000000000002220 ) ;
#7089=VERTEX_POINT ( 'NONE', #6469 ) ;
#7102=CARTESIAN_POINT ( 'NONE',  ( 44.62907851819101523, 71.79144999128007498, 25.00000000000000000 ) ) ;
#7113=EDGE_LOOP ( 'NONE', ( #7218, #7909, #158, #8950 ) ) ;
#7114=CARTESIAN_POINT ( 'NONE',  ( 46.97979101891770171, 52.38859998837343568, 25.00000000000000000 ) ) ;
#7148=CIRCLE ( 'NONE', #9512, 2.500000000000002220 ) ;
#7153=EDGE_CURVE ( 'NONE', #192, #3729, #4593, .T. ) ;
#7158=VECTOR ( 'NONE', #10284, 1000.000000000000000 ) ;
#7161=EDGE_CURVE ( 'NONE', #13574, #4466, #8140, .T. ) ;
#7162=ORIENTED_EDGE ( 'NONE', *, *, #2244, .T. ) ;
#7164=VERTEX_POINT ( 'NONE', #5865 ) ;
#7165=AXIS2_PLACEMENT_3D ( 'NONE', #13591, #10198, #184 ) ;
#7187=ORIENTED_EDGE ( 'NONE', *, *, #7762, .F. ) ;
#7202=ORIENTED_EDGE ( 'NONE', *, *, #3686, .F. ) ;
#7209=LINE ( 'NONE', #494, #7630 ) ;
#7217=ORIENTED_EDGE ( 'NONE', *, *, #2543, .F. ) ;
#7218=ORIENTED_EDGE ( 'NONE', *, *, #7698, .T. ) ;
#7222=DIRECTION ( 'NONE',  ( -1.000000000000000000, 0.000000000000000000, 0.000000000000000000 ) ) ;
#7223=AXIS2_PLACEMENT_3D ( 'NONE', #6418, #12131, #4178 ) ;
#7224=CARTESIAN_POINT ( 'NONE',  ( 56.83050351964436686, 32.98574998546678927, 25.00000000000000000 ) ) ;
#7243=DIRECTION ( 'NONE',  ( 0.000000000000000000, 0.000000000000000000, -1.000000000000000000 ) ) ;
#7248=ADVANCED_FACE ( 'NONE', ( #257 ), #5721, .T. ) ;
#7250=ORIENTED_EDGE ( 'NONE', *, *, #10086, .T. ) ;
#7261=PLANE ( 'NONE',  #138 ) ;
#7314=AXIS2_PLACEMENT_3D ( 'NONE', #12938, #9761, #14240 ) ;
#7321=EDGE_LOOP ( 'NONE', ( #2598, #7918, #13930, #3894 ) ) ;
#7327=CARTESIAN_POINT ( 'NONE',  ( 21.68170757442808849, 141.2731697022877313, 25.00000000000000000 ) ) ;
#7341=ORIENTED_EDGE ( 'NONE', *, *, #11807, .F. ) ;
#7352=FACE_BOUND ( 'NONE', #6893, .T. ) ;
#7367=EDGE_CURVE ( 'NONE', #5200, #45, #11745, .T. ) ;
#7370=ORIENTED_EDGE ( 'NONE', *, *, #11403, .T. ) ;
#7372=ORIENTED_EDGE ( 'NONE', *, *, #13842, .T. ) ;
#7379=CARTESIAN_POINT ( 'NONE',  ( 61.68121602037100359, 13.58289998256015352, 25.00000000000000000 ) ) ;
#7380=DIRECTION ( 'NONE',  ( -1.000000000000000000, 0.000000000000000000, 0.000000000000000000 ) ) ;
#7383=DIRECTION ( 'NONE',  ( -1.000000000000000000, 0.000000000000000000, 0.000000000000000000 ) ) ;
#7387=CARTESIAN_POINT ( 'NONE',  ( 44.55443476855437268, 62.09002498982675888, 25.00000000000000000 ) ) ;
#7395=VECTOR ( 'NONE', #9538, 1000.000000000000114 ) ;
#7399=DIRECTION ( 'NONE',  ( 0.000000000000000000, 0.000000000000000000, -1.000000000000000000 ) ) ;
#7411=ORIENTED_EDGE ( 'NONE', *, *, #6384, .T. ) ;
#7428=AXIS2_PLACEMENT_3D ( 'NONE', #385, #1193, #3680 ) ;
#7445=CYLINDRICAL_SURFACE ( 'NONE', #11720, 2.500000000000002220 ) ;
#7453=EDGE_LOOP ( 'NONE', ( #11721, #2031 ) ) ;
#7454=DIRECTION ( 'NONE',  ( -1.000000000000000000, 0.000000000000000000, 0.000000000000000000 ) ) ;
#7460=CARTESIAN_POINT ( 'NONE',  ( 34.92765351673772045, 110.5971499970933536, -25.00000000000000000 ) ) ;
#7462=ORIENTED_EDGE ( 'NONE', *, *, #3613, .F. ) ;
#7470=DIRECTION ( 'NONE',  ( 1.000000000000000000, 0.000000000000000000, 0.000000000000000000 ) ) ;
#7478=EDGE_CURVE ( 'NONE', #1985, #3428, #6946, .T. ) ;
#7482=CIRCLE ( 'NONE', #8890, 2.500000000000002220 ) ;
#7483=COLOUR_RGB ( '', 0.08235294, 0.09019608, 0.10196078) ;
#7488=VECTOR ( 'NONE', #9559, 1000.000000000000000 ) ;
#7491=CARTESIAN_POINT ( 'NONE',  ( 61.53192852109764743, -5.819950020346492892, 25.00000000000000000 ) ) ;
#7492=DIRECTION ( 'NONE',  ( -1.000000000000000000, 0.000000000000000000, 0.000000000000000000 ) ) ;
#7500=EDGE_LOOP ( 'NONE', ( #833, #3712, #1195, #8893 ) ) ;
#7502=VERTEX_POINT ( 'NONE', #3186 ) ;
#7509=VECTOR ( 'NONE', #9752, 1000.000000000000000 ) ;
#7520=VECTOR ( 'NONE', #1180, 1000.000000000000000 ) ;
#7521=CARTESIAN_POINT ( 'NONE',  ( 37.35300976710104948, 100.8957249956400375, 25.00000000000000000 ) ) ;
#7522=EDGE_CURVE ( 'NONE', #4685, #2107, #3012, .T. ) ;
#7531=DIRECTION ( 'NONE',  ( 1.000000000000000000, 0.000000000000000000, 0.000000000000000000 ) ) ;
#7535=ORIENTED_EDGE ( 'NONE', *, *, #5206, .F. ) ;
#7545=DIRECTION ( 'NONE',  ( 1.000000000000000000, 0.000000000000000000, 0.000000000000000000 ) ) ;
#7552=VERTEX_POINT ( 'NONE', #1121 ) ;
#7553=CARTESIAN_POINT ( 'NONE',  ( 64.03192852109765454, -5.819950020346492892, -25.00000000000000000 ) ) ;
#7566=CARTESIAN_POINT ( 'NONE',  ( 59.10586122665984732, -20.42344490663941414, 35.00000000000000000 ) ) ;
#7568=CARTESIAN_POINT ( 'NONE',  ( 64.10657227073433262, 3.881474981106830757, 25.00000000000000000 ) ) ;
#7576=ORIENTED_EDGE ( 'NONE', *, *, #7161, .F. ) ;
#7600=VERTEX_POINT ( 'NONE', #896 ) ;
#7613=ADVANCED_FACE ( 'NONE', ( #1480 ), #13570, .T. ) ;
#7619=FACE_BOUND ( 'NONE', #1055, .T. ) ;
#7630=VECTOR ( 'NONE', #10588, 1000.000000000000000 ) ;
#7635=( NAMED_UNIT ( * ) SI_UNIT ( $, .STERADIAN. ) SOLID_ANGLE_UNIT ( ) );
#7636=CARTESIAN_POINT ( 'NONE',  ( 59.10586122665984732, -20.42344490663941414, 35.00000000000000000 ) ) ;
#7644=EDGE_LOOP ( 'NONE', ( #8775, #245, #8419, #14364 ) ) ;
#7656=DIRECTION ( 'NONE',  ( 0.000000000000000000, 0.000000000000000000, -1.000000000000000000 ) ) ;
#7657=ORIENTED_EDGE ( 'NONE', *, *, #1851, .F. ) ;
#7682=EDGE_CURVE ( 'NONE', #6682, #13714, #12808, .T. ) ;
#7687=CARTESIAN_POINT ( 'NONE',  ( 27.57694101601105530, 130.0000000000000000, -25.00000000000000000 ) ) ;
#7697=DIRECTION ( 'NONE',  ( 0.000000000000000000, 0.000000000000000000, -1.000000000000000000 ) ) ;
#7698=EDGE_CURVE ( 'NONE', #6127, #2739, #106, .T. ) ;
#7715=EDGE_CURVE ( 'NONE', #10509, #12288, #13760, .T. ) ;
#7718=FILL_AREA_STYLE_COLOUR ( '', #7483 ) ;
#7720=EDGE_CURVE ( 'NONE', #3991, #4685, #10552, .T. ) ;
#7725=ORIENTED_EDGE ( 'NONE', *, *, #13188, .F. ) ;
#7729=FACE_OUTER_BOUND ( 'NONE', #8267, .T. ) ;
#7733=CARTESIAN_POINT ( 'NONE',  ( 59.10586122665984732, -20.42344490663941414, -35.00000000000000000 ) ) ;
#7740=VERTEX_POINT ( 'NONE', #684 ) ;
#7762=EDGE_CURVE ( 'NONE', #7552, #6880, #2808, .T. ) ;
#7767=ORIENTED_EDGE ( 'NONE', *, *, #9715, .T. ) ;
#7772=DIRECTION ( 'NONE',  ( -1.000000000000000000, 0.000000000000000000, 0.000000000000000000 ) ) ;
#7795=DIRECTION ( 'NONE',  ( 1.000000000000000000, 0.000000000000000000, 0.000000000000000000 ) ) ;
#7803=EDGE_CURVE ( 'NONE', #3245, #1176, #5134, .T. ) ;
#7809=DIRECTION ( 'NONE',  ( 0.000000000000000000, 0.000000000000000000, -1.000000000000000000 ) ) ;
#7815=LINE ( 'NONE', #2046, #5440 ) ;
#7826=CARTESIAN_POINT ( 'NONE',  ( 62.10586122665984732, -20.42344490663941414, -23.00000000000000000 ) ) ;
#7829=ORIENTED_EDGE ( 'NONE', *, *, #3947, .F. ) ;
#7838=CARTESIAN_POINT ( 'NONE',  ( 59.10586122665984732, -20.42344490663941414, 35.00000000000000000 ) ) ;
#7852=LINE ( 'NONE', #11088, #677 ) ;
#7865=ORIENTED_EDGE ( 'NONE', *, *, #11473, .T. ) ;
#7880=AXIS2_PLACEMENT_3D ( 'NONE', #12542, #12691, #11520 ) ;
#7882=FACE_BOUND ( 'NONE', #9066, .T. ) ;
#7883=VERTEX_POINT ( 'NONE', #10030 ) ;
#7884=ADVANCED_FACE ( 'NONE', ( #5351 ), #13130, .T. ) ;
#7885=DIRECTION ( 'NONE',  ( 0.000000000000000000, 0.000000000000000000, -1.000000000000000000 ) ) ;
#7887=VECTOR ( 'NONE', #7243, 1000.000000000000000 ) ;
#7903=CARTESIAN_POINT ( 'NONE',  ( 31.38313257588138683, 143.6985259526510674, 25.00000000000000000 ) ) ;
#7904=ADVANCED_FACE ( 'NONE', ( #5422 ), #14220, .T. ) ;
#7905=AXIS2_PLACEMENT_3D ( 'NONE', #8816, #3066, #7492 ) ;
#7909=ORIENTED_EDGE ( 'NONE', *, *, #4211, .F. ) ;
#7912=VECTOR ( 'NONE', #7795, 1000.000000000000000 ) ;
#7918=ORIENTED_EDGE ( 'NONE', *, *, #4677, .T. ) ;
#7926=DIRECTION ( 'NONE',  ( 1.000000000000000000, 0.000000000000000000, 0.000000000000000000 ) ) ;
#7942=ORIENTED_EDGE ( 'NONE', *, *, #2729, .F. ) ;
#7947=DIRECTION ( 'NONE',  ( 0.000000000000000000, 0.000000000000000000, -1.000000000000000000 ) ) ;
#7954=ORIENTED_EDGE ( 'NONE', *, *, #5206, .T. ) ;
#7963=ORIENTED_EDGE ( 'NONE', *, *, #8528, .T. ) ;
#7966=CARTESIAN_POINT ( 'NONE',  ( 71.80728622811317052, -17.99808865627607801, -25.00000000000000000 ) ) ;
#7968=ADVANCED_FACE ( 'NONE', ( #1925 ), #8642, .F. ) ;
#7973=DIRECTION ( 'NONE',  ( 0.000000000000000000, 0.000000000000000000, -1.000000000000000000 ) ) ;
#7976=FACE_OUTER_BOUND ( 'NONE', #7321, .T. ) ;
#7979=ADVANCED_FACE ( 'NONE', ( #10843 ), #10905, .T. ) ;
#7981=AXIS2_PLACEMENT_3D ( 'NONE', #828, #3048, #7470 ) ;
#7988=AXIS2_PLACEMENT_3D ( 'NONE', #7521, #8328, #8490 ) ;
#7998=AXIS2_PLACEMENT_3D ( 'NONE', #5578, #10122, #1058 ) ;
#8002=CARTESIAN_POINT ( 'NONE',  ( 35.00229726637439143, 120.2985749985466839, 25.00000000000000000 ) ) ;
#8004=FACE_OUTER_BOUND ( 'NONE', #2962, .T. ) ;
#8009=DIRECTION ( 'NONE',  ( 1.000000000000000000, 0.000000000000000000, 0.000000000000000000 ) ) ;
#8015=VECTOR ( 'NONE', #12565, 1000.000000000000000 ) ;
#8016=LINE ( 'NONE', #3431, #7158 ) ;
#8041=DIRECTION ( 'NONE',  ( 0.000000000000000000, 0.000000000000000000, -1.000000000000000000 ) ) ;
#8043=VERTEX_POINT ( 'NONE', #7903 ) ;
#8046=PLANE ( 'NONE',  #5405 ) ;
#8047=ORIENTED_EDGE ( 'NONE', *, *, #3284, .F. ) ;
#8057=CARTESIAN_POINT ( 'NONE',  ( 47.12907851819101523, 71.79144999128007498, 25.00000000000000000 ) ) ;
#8066=ORIENTED_EDGE ( 'NONE', *, *, #11056, .F. ) ;
#8101=DIRECTION ( 'NONE',  ( -0.2425356250363329969, 0.9701425001453318764, -9.251858538542973800E-15 ) ) ;
#8106=VERTEX_POINT ( 'NONE', #6040 ) ;
#8140=LINE ( 'NONE', #13515, #14014 ) ;
#8152=DIRECTION ( 'NONE',  ( 0.2425356250363327748, -0.9701425001453319874, -0.000000000000000000 ) ) ;
#8161=FACE_OUTER_BOUND ( 'NONE', #12344, .T. ) ;
#8174=CARTESIAN_POINT ( 'NONE',  ( 27.57694101601105530, 130.0000000000000000, 25.00000000000000000 ) ) ;
#8176=LINE ( 'NONE', #11622, #9085 ) ;
#8186=CARTESIAN_POINT ( 'NONE',  ( 18.68170757442808849, 141.2731697022877313, -35.00000000000000000 ) ) ;
#8193=CARTESIAN_POINT ( 'NONE',  ( 71.80728622811317052, -17.99808865627607801, -28.00000000000000000 ) ) ;
#8194=ADVANCED_FACE ( 'NONE', ( #13170 ), #793, .T. ) ;
#8197=AXIS2_PLACEMENT_3D ( 'NONE', #1532, #2417, #11477 ) ;
#8200=EDGE_LOOP ( 'NONE', ( #10266, #1567 ) ) ;
#8217=( GEOMETRIC_REPRESENTATION_CONTEXT ( 3 ) GLOBAL_UNCERTAINTY_ASSIGNED_CONTEXT ( ( #4138 ) ) GLOBAL_UNIT_ASSIGNED_CONTEXT ( ( #5511, #6676, #10132 ) ) REPRESENTATION_CONTEXT ( 'NONE', 'WORKASPACE' ) );
#8233=DIRECTION ( 'NONE',  ( -0.000000000000000000, -0.000000000000000000, -1.000000000000000000 ) ) ;
#8236=CARTESIAN_POINT ( 'NONE',  ( 39.77836601746437850, 91.19429999418670718, 25.00000000000000000 ) ) ;
#8238=FACE_OUTER_BOUND ( 'NONE', #903, .T. ) ;
#8247=ORIENTED_EDGE ( 'NONE', *, *, #4663, .F. ) ;
#8253=LINE ( 'NONE', #13495, #4886 ) ;
#8254=CARTESIAN_POINT ( 'NONE',  ( 42.27836601746437850, 91.19429999418670718, 25.00000000000000000 ) ) ;
#8259=AXIS2_PLACEMENT_3D ( 'NONE', #9257, #12618, #490 ) ;
#8260=LINE ( 'NONE', #9214, #3341 ) ;
#8263=EDGE_LOOP ( 'NONE', ( #3658, #10324 ) ) ;
#8267=EDGE_LOOP ( 'NONE', ( #2826, #8612, #4193, #7217 ) ) ;
#8279=DIRECTION ( 'NONE',  ( 0.000000000000000000, 0.000000000000000000, 1.000000000000000000 ) ) ;
#8293=FACE_BOUND ( 'NONE', #6888, .T. ) ;
#8297=CARTESIAN_POINT ( 'NONE',  ( 59.10586122665984732, -20.42344490663941414, 35.00000000000000000 ) ) ;
#8319=DIRECTION ( 'NONE',  ( -1.000000000000000000, 0.000000000000000000, 0.000000000000000000 ) ) ;
#8328=DIRECTION ( 'NONE',  ( -0.000000000000000000, -0.000000000000000000, -1.000000000000000000 ) ) ;
#8335=PLANE ( 'NONE',  #4057 ) ;
#8350=CARTESIAN_POINT ( 'NONE',  ( 21.68170757442808849, 141.2731697022877313, 23.00000000000000000 ) ) ;
#8353=VECTOR ( 'NONE', #2656, 1000.000000000000000 ) ;
#8355=CIRCLE ( 'NONE', #4192, 2.500000000000002220 ) ;
#8360=PLANE ( 'NONE',  #12784 ) ;
#8408=LINE ( 'NONE', #5119, #6828 ) ;
#8417=ADVANCED_FACE ( 'NONE', ( #8004 ), #482, .T. ) ;
#8419=ORIENTED_EDGE ( 'NONE', *, *, #3583, .T. ) ;
#8426=AXIS2_PLACEMENT_3D ( 'NONE', #689, #13059, #6514 ) ;
#8428=VECTOR ( 'NONE', #5043, 1000.000000000000000 ) ;
#8430=CARTESIAN_POINT ( 'NONE',  ( 0.000000000000000000, 0.000000000000000000, -35.00000000000000000 ) ) ;
#8435=STYLED_ITEM ( 'NONE', ( #2246 ), #11686 ) ;
#8445=DIRECTION ( 'NONE',  ( 0.2425356250363327471, -0.9701425001453319874, -0.000000000000000000 ) ) ;
#8460=CIRCLE ( 'NONE', #10807, 2.500000000000002220 ) ;
#8468=DIRECTION ( 'NONE',  ( -0.000000000000000000, -0.000000000000000000, -1.000000000000000000 ) ) ;
#8476=VECTOR ( 'NONE', #13412, 1000.000000000000000 ) ;
#8477=ORIENTED_EDGE ( 'NONE', *, *, #7153, .T. ) ;
#8490=DIRECTION ( 'NONE',  ( 1.000000000000000000, 0.000000000000000000, 0.000000000000000000 ) ) ;
#8492=ORIENTED_EDGE ( 'NONE', *, *, #12937, .T. ) ;
#8494=EDGE_LOOP ( 'NONE', ( #2950, #14007 ) ) ;
#8498=AXIS2_PLACEMENT_3D ( 'NONE', #4174, #6477, #4112 ) ;
#8504=ORIENTED_EDGE ( 'NONE', *, *, #9227, .T. ) ;
#8511=ADVANCED_FACE ( 'NONE', ( #3188 ), #1725, .F. ) ;
#8525=DIRECTION ( 'NONE',  ( 1.000000000000000000, 0.000000000000000000, 0.000000000000000000 ) ) ;
#8527=ORIENTED_EDGE ( 'NONE', *, *, #3243, .F. ) ;
#8528=EDGE_CURVE ( 'NONE', #4078, #12827, #4840, .T. ) ;
#8545=VERTEX_POINT ( 'NONE', #11751 ) ;
#8552=AXIS2_PLACEMENT_3D ( 'NONE', #9001, #6665, #5567 ) ;
#8557=EDGE_CURVE ( 'NONE', #11484, #5967, #1646, .T. ) ;
#8572=ORIENTED_EDGE ( 'NONE', *, *, #11196, .T. ) ;
#8573=FACE_OUTER_BOUND ( 'NONE', #6953, .T. ) ;
#8591=ORIENTED_EDGE ( 'NONE', *, *, #150, .T. ) ;
#8612=ORIENTED_EDGE ( 'NONE', *, *, #6831, .T. ) ;
#8614=DIRECTION ( 'NONE',  ( -0.2425356250363330801, 0.9701425001453319874, 0.000000000000000000 ) ) ;
#8638=DIRECTION ( 'NONE',  ( -0.9701425001453318764, -0.2425356250363329969, 0.000000000000000000 ) ) ;
#8642=PLANE ( 'NONE',  #1349 ) ;
#8644=CARTESIAN_POINT ( 'NONE',  ( 18.68170757442808849, 141.2731697022877313, -35.00000000000000000 ) ) ;
#8645=CIRCLE ( 'NONE', #4475, 2.500000000000002220 ) ;
#8646=EDGE_CURVE ( 'NONE', #1328, #8838, #11612, .T. ) ;
#8665=FACE_BOUND ( 'NONE', #3830, .T. ) ;
#8686=EDGE_LOOP ( 'NONE', ( #5124, #2676, #5789, #6851 ) ) ;
#8689=ORIENTED_EDGE ( 'NONE', *, *, #11936, .F. ) ;
#8692=AXIS2_PLACEMENT_3D ( 'NONE', #11558, #11287, #13496 ) ;
#8701=AXIS2_PLACEMENT_3D ( 'NONE', #4585, #9016, #5519 ) ;
#8714=ORIENTED_EDGE ( 'NONE', *, *, #1819, .F. ) ;
#8731=ORIENTED_EDGE ( 'NONE', *, *, #13325, .T. ) ;
#8739=DIRECTION ( 'NONE',  ( 0.000000000000000000, 0.000000000000000000, -1.000000000000000000 ) ) ;
#8744=DIRECTION ( 'NONE',  ( 0.000000000000000000, 0.000000000000000000, -1.000000000000000000 ) ) ;
#8752=EDGE_CURVE ( 'NONE', #3420, #4122, #3653, .T. ) ;
#8775=ORIENTED_EDGE ( 'NONE', *, *, #2503, .F. ) ;
#8792=CARTESIAN_POINT ( 'NONE',  ( 30.07694101601105530, 130.0000000000000000, 25.00000000000000000 ) ) ;
#8799=CIRCLE ( 'NONE', #4386, 2.500000000000002220 ) ;
#8804=ORIENTED_EDGE ( 'NONE', *, *, #4368, .T. ) ;
#8816=CARTESIAN_POINT ( 'NONE',  ( 49.47979101891770171, 52.38859998837343568, 25.00000000000000000 ) ) ;
#8820=VECTOR ( 'NONE', #2522, 1000.000000000000000 ) ;
#8833=VECTOR ( 'NONE', #5523, 1000.000000000000000 ) ;
#8838=VERTEX_POINT ( 'NONE', #4018 ) ;
#8841=CIRCLE ( 'NONE', #9074, 2.500000000000002220 ) ;
#8842=ORIENTED_EDGE ( 'NONE', *, *, #6189, .F. ) ;
#8843=ORIENTED_EDGE ( 'NONE', *, *, #367, .T. ) ;
#8852=CARTESIAN_POINT ( 'NONE',  ( 31.38313257588138683, 143.6985259526510390, -28.00000000000000000 ) ) ;
#8857=CARTESIAN_POINT ( 'NONE',  ( 59.18121602037099649, 13.58289998256015352, 25.00000000000000000 ) ) ;
#8859=ADVANCED_FACE ( 'NONE', ( #4241 ), #6114, .T. ) ;
#8872=CARTESIAN_POINT ( 'NONE',  ( 18.68170757442808849, 141.2731697022877313, -23.00000000000000000 ) ) ;
#8873=ORIENTED_EDGE ( 'NONE', *, *, #4600, .T. ) ;
#8890=AXIS2_PLACEMENT_3D ( 'NONE', #1991, #14216, #7531 ) ;
#8893=ORIENTED_EDGE ( 'NONE', *, *, #4971, .F. ) ;
#8897=EDGE_LOOP ( 'NONE', ( #7187, #6028, #10275, #877 ) ) ;
#8905=LINE ( 'NONE', #11175, #14078 ) ;
#8913=CIRCLE ( 'NONE', #12912, 2.500000000000002220 ) ;
#8916=VERTEX_POINT ( 'NONE', #11842 ) ;
#8919=DIRECTION ( 'NONE',  ( -1.000000000000000000, 0.000000000000000000, 0.000000000000000000 ) ) ;
#8934=CIRCLE ( 'NONE', #7998, 2.500000000000002220 ) ;
#8943=CIRCLE ( 'NONE', #4535, 2.500000000000002220 ) ;
#8950=ORIENTED_EDGE ( 'NONE', *, *, #12096, .T. ) ;
#8952=DIRECTION ( 'NONE',  ( 0.000000000000000000, 0.000000000000000000, -1.000000000000000000 ) ) ;
#8968=ORIENTED_EDGE ( 'NONE', *, *, #13189, .F. ) ;
#8982=ORIENTED_EDGE ( 'NONE', *, *, #3008, .F. ) ;
#8983=EDGE_LOOP ( 'NONE', ( #8066, #8047 ) ) ;
#8996=ORIENTED_EDGE ( 'NONE', *, *, #7698, .F. ) ;
#9001=CARTESIAN_POINT ( 'NONE',  ( 56.75585977000769589, 23.28432498401347672, -25.00000000000000000 ) ) ;
#9016=DIRECTION ( 'NONE',  ( 0.000000000000000000, 0.000000000000000000, -1.000000000000000000 ) ) ;
#9021=ORIENTED_EDGE ( 'NONE', *, *, #7803, .F. ) ;
#9022=DIRECTION ( 'NONE',  ( 1.000000000000000000, 0.000000000000000000, 0.000000000000000000 ) ) ;
#9054=ORIENTED_EDGE ( 'NONE', *, *, #3460, .T. ) ;
#9057=PLANE ( 'NONE',  #12410 ) ;
#9060=PLANE ( 'NONE',  #9116 ) ;
#9062=LINE ( 'NONE', #7, #1689 ) ;
#9066=EDGE_LOOP ( 'NONE', ( #2332, #11215 ) ) ;
#9074=AXIS2_PLACEMENT_3D ( 'NONE', #9186, #13683, #2542 ) ;
#9083=EDGE_LOOP ( 'NONE', ( #450, #5844 ) ) ;
#9085=VECTOR ( 'NONE', #6131, 1000.000000000000000 ) ;
#9087=UNCERTAINTY_MEASURE_WITH_UNIT (LENGTH_MEASURE( 1.000000000000000082E-05 ), #2368, 'distance_accuracy_value', 'NONE');
#9101=ORIENTED_EDGE ( 'NONE', *, *, #7720, .F. ) ;
#9107=CARTESIAN_POINT ( 'NONE',  ( 64.03192852109765454, -5.819950020346492892, -25.00000000000000000 ) ) ;
#9111=ORIENTED_EDGE ( 'NONE', *, *, #3613, .T. ) ;
#9113=DIRECTION ( 'NONE',  ( -1.000000000000000000, 0.000000000000000000, 0.000000000000000000 ) ) ;
#9116=AXIS2_PLACEMENT_3D ( 'NONE', #7079, #8101, #13629 ) ;
#9141=EDGE_CURVE ( 'NONE', #3184, #7502, #1976, .T. ) ;
#9144=EDGE_LOOP ( 'NONE', ( #14277, #7942 ) ) ;
#9171=ORIENTED_EDGE ( 'NONE', *, *, #4900, .F. ) ;
#9181=DIRECTION ( 'NONE',  ( 0.000000000000000000, 0.000000000000000000, -1.000000000000000000 ) ) ;
#9182=EDGE_LOOP ( 'NONE', ( #3450, #4982 ) ) ;
#9184=CIRCLE ( 'NONE', #561, 2.500000000000002220 ) ;
#9186=CARTESIAN_POINT ( 'NONE',  ( 49.47979101891770171, 52.38859998837343568, 25.00000000000000000 ) ) ;
#9202=ORIENTED_EDGE ( 'NONE', *, *, #5080, .T. ) ;
#9203=DIRECTION ( 'NONE',  ( -0.9701425001453318764, -0.2425356250363329969, 0.000000000000000000 ) ) ;
#9213=ORIENTED_EDGE ( 'NONE', *, *, #3008, .T. ) ;
#9214=CARTESIAN_POINT ( 'NONE',  ( 61.53192852109764743, -5.819950020346492892, 25.00000000000000000 ) ) ;
#9227=EDGE_CURVE ( 'NONE', #8545, #13907, #10369, .T. ) ;
#9233=ORIENTED_EDGE ( 'NONE', *, *, #11083, .T. ) ;
#9240=CARTESIAN_POINT ( 'NONE',  ( 71.80728622811317052, -17.99808865627607801, -25.00000000000000000 ) ) ;
#9257=CARTESIAN_POINT ( 'NONE',  ( 42.20372226782770753, 81.49287499273339108, 25.00000000000000000 ) ) ;
#9261=DIRECTION ( 'NONE',  ( -1.000000000000000000, 0.000000000000000000, 0.000000000000000000 ) ) ;
#9265=CARTESIAN_POINT ( 'NONE',  ( 61.60657227073433262, 3.881474981106830313, 25.00000000000000000 ) ) ;
#9268=AXIS2_PLACEMENT_3D ( 'NONE', #6308, #2966, #8279 ) ;
#9272=ORIENTED_EDGE ( 'NONE', *, *, #3842, .F. ) ;
#9286=AXIS2_PLACEMENT_3D ( 'NONE', #10997, #8739, #6528 ) ;
#9293=ORIENTED_EDGE ( 'NONE', *, *, #5383, .T. ) ;
#9301=VECTOR ( 'NONE', #4133, 999.9999999999998863 ) ;
#9345=VECTOR ( 'NONE', #6048, 999.9999999999998863 ) ;
#9377=EDGE_LOOP ( 'NONE', ( #5445, #13705 ) ) ;
#9379=DIRECTION ( 'NONE',  ( 0.000000000000000000, 0.000000000000000000, 1.000000000000000000 ) ) ;
#9386=CIRCLE ( 'NONE', #8692, 2.500000000000002220 ) ;
#9400=VERTEX_POINT ( 'NONE', #10592 ) ;
#9404=ORIENTED_EDGE ( 'NONE', *, *, #9773, .T. ) ;
#9408=CARTESIAN_POINT ( 'NONE',  ( 59.10586122665984732, -20.42344490663941414, -35.00000000000000000 ) ) ;
#9419=ADVANCED_FACE ( 'NONE', ( #4016 ), #4877, .T. ) ;
#9428=CARTESIAN_POINT ( 'NONE',  ( 71.80728622811317052, -17.99808865627607801, -28.00000000000000000 ) ) ;
#9434=CARTESIAN_POINT ( 'NONE',  ( 21.68170757442808849, 141.2731697022877313, -35.00000000000000000 ) ) ;
#9442=CARTESIAN_POINT ( 'NONE',  ( 32.42765351673771335, 110.5971499970933536, 25.00000000000000000 ) ) ;
#9447=ADVANCED_FACE ( 'NONE', ( #12053 ), #2024, .T. ) ;
#9456=ORIENTED_EDGE ( 'NONE', *, *, #674, .F. ) ;
#9465=CARTESIAN_POINT ( 'NONE',  ( 21.68170757442806362, 141.2731697022877313, 25.00000000000000000 ) ) ;
#9468=CARTESIAN_POINT ( 'NONE',  ( 18.68170757442808849, 141.2731697022877313, 35.00000000000000000 ) ) ;
#9504=ORIENTED_EDGE ( 'NONE', *, *, #2982, .F. ) ;
#9509=CARTESIAN_POINT ( 'NONE',  ( 59.25585977000769589, 23.28432498401347672, -25.00000000000000000 ) ) ;
#9512=AXIS2_PLACEMENT_3D ( 'NONE', #13936, #3909, #7772 ) ;
#9520=EDGE_CURVE ( 'NONE', #4078, #13851, #11010, .T. ) ;
#9526=ORIENTED_EDGE ( 'NONE', *, *, #418, .F. ) ;
#9537=DIRECTION ( 'NONE',  ( 1.000000000000000000, 0.000000000000000000, 0.000000000000000000 ) ) ;
#9538=DIRECTION ( 'NONE',  ( -0.9701425001453318764, -0.2425356250363329969, 0.000000000000000000 ) ) ;
#9548=DIRECTION ( 'NONE',  ( 0.000000000000000000, 0.000000000000000000, -1.000000000000000000 ) ) ;
#9559=DIRECTION ( 'NONE',  ( 0.000000000000000000, 0.000000000000000000, -1.000000000000000000 ) ) ;
#9562=CARTESIAN_POINT ( 'NONE',  ( 21.68170757442808849, 141.2731697022877313, -25.00000000000000000 ) ) ;
#9570=VECTOR ( 'NONE', #635, 1000.000000000000000 ) ;
#9597=EDGE_LOOP ( 'NONE', ( #1280, #1972 ) ) ;
#9611=DIRECTION ( 'NONE',  ( 0.000000000000000000, 0.000000000000000000, 1.000000000000000000 ) ) ;
#9621=ORIENTED_EDGE ( 'NONE', *, *, #4600, .F. ) ;
#9634=AXIS2_PLACEMENT_3D ( 'NONE', #9408, #13676, #9181 ) ;
#9640=DIRECTION ( 'NONE',  ( 0.000000000000000000, 0.000000000000000000, 1.000000000000000000 ) ) ;
#9646=VECTOR ( 'NONE', #4754, 1000.000000000000000 ) ;
#9660=CARTESIAN_POINT ( 'NONE',  ( 61.60657227073433262, 3.881474981106830313, -25.00000000000000000 ) ) ;
#9661=AXIS2_PLACEMENT_3D ( 'NONE', #5161, #14108, #11356 ) ;
#9675=DIRECTION ( 'NONE',  ( 0.000000000000000000, 0.000000000000000000, -1.000000000000000000 ) ) ;
#9680=ORIENTED_EDGE ( 'NONE', *, *, #10352, .F. ) ;
#9688=EDGE_CURVE ( 'NONE', #13851, #13075, #8355, .T. ) ;
#9715=EDGE_CURVE ( 'NONE', #10016, #4769, #6265, .T. ) ;
#9722=CYLINDRICAL_SURFACE ( 'NONE', #7223, 2.500000000000002220 ) ;
#9731=PRODUCT_DEFINITION ( 'UNKNOWN', '', #2915, #14371 ) ;
#9741=CARTESIAN_POINT ( 'NONE',  ( 31.38313257588138683, 143.6985259526510390, 28.00000000000000000 ) ) ;
#9752=DIRECTION ( 'NONE',  ( 0.000000000000000000, 0.000000000000000000, -1.000000000000000000 ) ) ;
#9757=DIRECTION ( 'NONE',  ( 1.000000000000000000, 0.000000000000000000, 0.000000000000000000 ) ) ;
#9759=EDGE_LOOP ( 'NONE', ( #12502, #4030, #1609, #1735 ) ) ;
#9761=DIRECTION ( 'NONE',  ( -0.000000000000000000, -0.000000000000000000, -1.000000000000000000 ) ) ;
#9762=AXIS2_PLACEMENT_3D ( 'NONE', #9741, #11060, #4204 ) ;
#9768=ORIENTED_EDGE ( 'NONE', *, *, #4971, .T. ) ;
#9771=FACE_OUTER_BOUND ( 'NONE', #13174, .T. ) ;
#9773=EDGE_CURVE ( 'NONE', #11937, #5807, #10932, .T. ) ;
#9803=CARTESIAN_POINT ( 'NONE',  ( 62.10586122665984732, -20.42344490663941414, 23.00000000000000000 ) ) ;
#9812=DIRECTION ( 'NONE',  ( -1.000000000000000000, 0.000000000000000000, 0.000000000000000000 ) ) ;
#9834=FACE_BOUND ( 'NONE', #13882, .T. ) ;
#9835=ORIENTED_EDGE ( 'NONE', *, *, #3267, .T. ) ;
#9839=ORIENTED_EDGE ( 'NONE', *, *, #7682, .F. ) ;
#9852=EDGE_CURVE ( 'NONE', #5618, #45, #6171, .T. ) ;
#9854=CIRCLE ( 'NONE', #3553, 2.500000000000002220 ) ;
#9862=DIRECTION ( 'NONE',  ( -1.000000000000000000, 0.000000000000000000, 0.000000000000000000 ) ) ;
#9877=ORIENTED_EDGE ( 'NONE', *, *, #1453, .T. ) ;
#9880=VECTOR ( 'NONE', #3733, 1000.000000000000000 ) ;
#9909=( NAMED_UNIT ( * ) SI_UNIT ( $, .STERADIAN. ) SOLID_ANGLE_UNIT ( ) );
#9914=FACE_BOUND ( 'NONE', #9144, .T. ) ;
#9916=EDGE_CURVE ( 'NONE', #13539, #5373, #4216, .T. ) ;
#9931=VERTEX_POINT ( 'NONE', #14164 ) ;
#9937=CARTESIAN_POINT ( 'NONE',  ( 56.83050351964436686, 32.98574998546678927, 25.00000000000000000 ) ) ;
#9940=DIRECTION ( 'NONE',  ( 0.000000000000000000, 0.000000000000000000, -1.000000000000000000 ) ) ;
#9943=ORIENTED_EDGE ( 'NONE', *, *, #11083, .F. ) ;
#9963=DIRECTION ( 'NONE',  ( 0.000000000000000000, 0.000000000000000000, -1.000000000000000000 ) ) ;
#9971=DIRECTION ( 'NONE',  ( 0.000000000000000000, 0.000000000000000000, -1.000000000000000000 ) ) ;
#9974=ADVANCED_FACE ( 'NONE', ( #3183 ), #10716, .T. ) ;
#9977=AXIS2_PLACEMENT_3D ( 'NONE', #3388, #2274, #11190 ) ;
#10000=EDGE_LOOP ( 'NONE', ( #6252, #12504, #6020, #8247 ) ) ;
#10001=DIRECTION ( 'NONE',  ( -1.000000000000000000, 0.000000000000000000, 0.000000000000000000 ) ) ;
#10006=FACE_OUTER_BOUND ( 'NONE', #1846, .T. ) ;
#10016=VERTEX_POINT ( 'NONE', #12035 ) ;
#10018=ORIENTED_EDGE ( 'NONE', *, *, #4337, .F. ) ;
#10030=CARTESIAN_POINT ( 'NONE',  ( 32.57694101601105530, 130.0000000000000000, 25.00000000000000000 ) ) ;
#10036=EDGE_CURVE ( 'NONE', #7552, #11916, #51, .T. ) ;
#10037=AXIS2_PLACEMENT_3D ( 'NONE', #10076, #6703, #11172 ) ;
#10052=ORIENTED_EDGE ( 'NONE', *, *, #12291, .T. ) ;
#10066=VECTOR ( 'NONE', #2520, 1000.000000000000000 ) ;
#10070=CIRCLE ( 'NONE', #13125, 2.500000000000002220 ) ;
#10073=ORIENTED_EDGE ( 'NONE', *, *, #685, .F. ) ;
#10076=CARTESIAN_POINT ( 'NONE',  ( 21.68170757442808849, 141.2731697022877313, -23.00000000000000000 ) ) ;
#10085=EDGE_LOOP ( 'NONE', ( #12414, #9877, #5121, #8968 ) ) ;
#10086=EDGE_CURVE ( 'NONE', #8838, #1328, #9386, .T. ) ;
#10087=AXIS2_PLACEMENT_3D ( 'NONE', #5475, #6709, #4474 ) ;
#10101=VERTEX_POINT ( 'NONE', #1050 ) ;
#10105=FACE_OUTER_BOUND ( 'NONE', #10000, .T. ) ;
#10116=AXIS2_PLACEMENT_3D ( 'NONE', #6961, #12469, #4716 ) ;
#10122=DIRECTION ( 'NONE',  ( 0.000000000000000000, 0.000000000000000000, -1.000000000000000000 ) ) ;
#10123=CIRCLE ( 'NONE', #319, 2.500000000000002220 ) ;
#10126=ORIENTED_EDGE ( 'NONE', *, *, #11936, .T. ) ;
#10128=FACE_OUTER_BOUND ( 'NONE', #4643, .T. ) ;
#10132=( NAMED_UNIT ( * ) SI_UNIT ( $, .STERADIAN. ) SOLID_ANGLE_UNIT ( ) );
#10143=CARTESIAN_POINT ( 'NONE',  ( 59.25585977000769589, 23.28432498401347672, 25.00000000000000000 ) ) ;
#10158=DIRECTION ( 'NONE',  ( -1.000000000000000000, 0.000000000000000000, 0.000000000000000000 ) ) ;
#10184=DIRECTION ( 'NONE',  ( -1.000000000000000000, 0.000000000000000000, 0.000000000000000000 ) ) ;
#10198=DIRECTION ( 'NONE',  ( 0.000000000000000000, 0.000000000000000000, -1.000000000000000000 ) ) ;
#10208=CARTESIAN_POINT ( 'NONE',  ( 30.07694101601105530, 130.0000000000000000, 25.00000000000000000 ) ) ;
#10210=ORIENTED_EDGE ( 'NONE', *, *, #8752, .F. ) ;
#10213=LINE ( 'NONE', #2257, #11420 ) ;
#10248=ORIENTED_EDGE ( 'NONE', *, *, #10625, .T. ) ;
#10260=DIRECTION ( 'NONE',  ( 0.000000000000000000, 0.000000000000000000, -1.000000000000000000 ) ) ;
#10266=ORIENTED_EDGE ( 'NONE', *, *, #1431, .T. ) ;
#10267=CARTESIAN_POINT ( 'NONE',  ( 59.18121602037099649, 13.58289998256015352, 25.00000000000000000 ) ) ;
#10274=ORIENTED_EDGE ( 'NONE', *, *, #3947, .T. ) ;
#10275=ORIENTED_EDGE ( 'NONE', *, *, #2392, .T. ) ;
#10279=AXIS2_PLACEMENT_3D ( 'NONE', #9107, #5882, #10365 ) ;
#10284=DIRECTION ( 'NONE',  ( 1.000000000000000000, 0.000000000000000000, 0.000000000000000000 ) ) ;
#10289=DIRECTION ( 'NONE',  ( 1.000000000000000000, 0.000000000000000000, 0.000000000000000000 ) ) ;
#10292=VECTOR ( 'NONE', #13749, 999.9999999999998863 ) ;
#10294=AXIS2_PLACEMENT_3D ( 'NONE', #10267, #11307, #9022 ) ;
#10302=CARTESIAN_POINT ( 'NONE',  ( 47.05443476855437268, 62.09002498982675888, -25.00000000000000000 ) ) ;
#10304=CIRCLE ( 'NONE', #12637, 2.500000000000002220 ) ;
#10313=CARTESIAN_POINT ( 'NONE',  ( 71.80728622811317052, -17.99808865627607801, 28.00000000000000000 ) ) ;
#10317=AXIS2_PLACEMENT_3D ( 'NONE', #14342, #4398, #2193 ) ;
#10323=ORIENTED_EDGE ( 'NONE', *, *, #5300, .F. ) ;
#10324=ORIENTED_EDGE ( 'NONE', *, *, #9715, .F. ) ;
#10340=CIRCLE ( 'NONE', #13406, 2.500000000000002220 ) ;
#10346=CARTESIAN_POINT ( 'NONE',  ( 44.55443476855437268, 62.09002498982675888, -25.00000000000000000 ) ) ;
#10352=EDGE_CURVE ( 'NONE', #12535, #696, #11461, .T. ) ;
#10365=DIRECTION ( 'NONE',  ( -1.000000000000000000, 0.000000000000000000, 0.000000000000000000 ) ) ;
#10369=LINE ( 'NONE', #5887, #436 ) ;
#10381=ORIENTED_EDGE ( 'NONE', *, *, #14154, .F. ) ;
#10387=FACE_OUTER_BOUND ( 'NONE', #7113, .T. ) ;
#10388=DIRECTION ( 'NONE',  ( -0.000000000000000000, -0.000000000000000000, -1.000000000000000000 ) ) ;
#10408=CARTESIAN_POINT ( 'NONE',  ( 47.12907851819101523, 71.79144999128007498, 25.00000000000000000 ) ) ;
#10415=DIRECTION ( 'NONE',  ( 1.000000000000000000, 0.000000000000000000, 0.000000000000000000 ) ) ;
#10438=VECTOR ( 'NONE', #14286, 1000.000000000000000 ) ;
#10447=CARTESIAN_POINT ( 'NONE',  ( 54.25585977000769589, 23.28432498401347672, -25.00000000000000000 ) ) ;
#10457=EDGE_CURVE ( 'NONE', #12827, #4078, #4480, .T. ) ;
#10463=AXIS2_PLACEMENT_3D ( 'NONE', #1275, #12188, #13295 ) ;
#10466=ORIENTED_EDGE ( 'NONE', *, *, #4090, .F. ) ;
#10468=ADVANCED_FACE ( 'NONE', ( #139 ), #280, .T. ) ;
#10471=LINE ( 'NONE', #2571, #13234 ) ;
#10472=CARTESIAN_POINT ( 'NONE',  ( 42.20372226782770753, 81.49287499273339108, -25.00000000000000000 ) ) ;
#10484=EDGE_CURVE ( 'NONE', #7883, #8838, #5032, .T. ) ;
#10495=ORIENTED_EDGE ( 'NONE', *, *, #5722, .T. ) ;
#10509=VERTEX_POINT ( 'NONE', #3801 ) ;
#10534=DIRECTION ( 'NONE',  ( 1.000000000000000000, 0.000000000000000000, 0.000000000000000000 ) ) ;
#10540=ADVANCED_FACE ( 'NONE', ( #8238 ), #11682, .T. ) ;
#10548=DIRECTION ( 'NONE',  ( -1.000000000000000000, 0.000000000000000000, 0.000000000000000000 ) ) ;
#10552=LINE ( 'NONE', #614, #8353 ) ;
#10565=ORIENTED_EDGE ( 'NONE', *, *, #14125, .T. ) ;
#10571=CARTESIAN_POINT ( 'NONE',  ( 62.10586122665984732, -20.42344490663941414, -35.00000000000000000 ) ) ;
#10578=FACE_BOUND ( 'NONE', #13739, .T. ) ;
#10588=DIRECTION ( 'NONE',  ( 0.000000000000000000, 0.000000000000000000, -1.000000000000000000 ) ) ;
#10592=CARTESIAN_POINT ( 'NONE',  ( 56.68121602037099649, 13.58289998256015352, -25.00000000000000000 ) ) ;
#10611=DIRECTION ( 'NONE',  ( 0.000000000000000000, 0.000000000000000000, -1.000000000000000000 ) ) ;
#10612=ORIENTED_EDGE ( 'NONE', *, *, #11418, .F. ) ;
#10624=CARTESIAN_POINT ( 'NONE',  ( 59.10586122665984732, -20.42344490663941414, 23.00000000000000000 ) ) ;
#10625=EDGE_CURVE ( 'NONE', #3362, #3826, #7482, .T. ) ;
#10639=ORIENTED_EDGE ( 'NONE', *, *, #7720, .T. ) ;
#10646=CARTESIAN_POINT ( 'NONE',  ( 62.10586122665987574, -20.42344490663940704, -25.00000000000000000 ) ) ;
#10651=DIRECTION ( 'NONE',  ( -0.9701425001453319874, -0.2425356250363327471, 0.000000000000000000 ) ) ;
#10655=CARTESIAN_POINT ( 'NONE',  ( 66.53192852109765454, -5.819950020346492892, 25.00000000000000000 ) ) ;
#10657=ORIENTED_EDGE ( 'NONE', *, *, #11056, .T. ) ;
#10693=AXIS2_PLACEMENT_3D ( 'NONE', #563, #3926, #8525 ) ;
#10705=CYLINDRICAL_SURFACE ( 'NONE', #8426, 2.500000000000002220 ) ;
#10716=CYLINDRICAL_SURFACE ( 'NONE', #979, 2.500000000000002220 ) ;
#10739=DIRECTION ( 'NONE',  ( 1.000000000000000000, 0.000000000000000000, 0.000000000000000000 ) ) ;
#10746=AXIS2_PLACEMENT_3D ( 'NONE', #13396, #12281, #2399 ) ;
#10751=PLANE ( 'NONE',  #1159 ) ;
#10757=CARTESIAN_POINT ( 'NONE',  ( 64.03192852109765454, -5.819950020346492892, 25.00000000000000000 ) ) ;
#10762=ADVANCED_FACE ( 'NONE', ( #10387 ), #9060, .T. ) ;
#10764=ORIENTED_EDGE ( 'NONE', *, *, #13189, .T. ) ;
#10765=CIRCLE ( 'NONE', #10279, 2.500000000000002220 ) ;
#10770=EDGE_LOOP ( 'NONE', ( #11546, #12343, #7576, #2028 ) ) ;
#10780=DIRECTION ( 'NONE',  ( 0.000000000000000000, 0.000000000000000000, 1.000000000000000000 ) ) ;
#10782=CARTESIAN_POINT ( 'NONE',  ( 39.70372226782770753, 81.49287499273339108, 25.00000000000000000 ) ) ;
#10790=ORIENTED_EDGE ( 'NONE', *, *, #11418, .T. ) ;
#10795=VECTOR ( 'NONE', #13819, 1000.000000000000000 ) ;
#10807=AXIS2_PLACEMENT_3D ( 'NONE', #6610, #8952, #12261 ) ;
#10843=FACE_OUTER_BOUND ( 'NONE', #12222, .T. ) ;
#10849=DIRECTION ( 'NONE',  ( -1.000000000000000000, 0.000000000000000000, 0.000000000000000000 ) ) ;
#10852=CARTESIAN_POINT ( 'NONE',  ( 62.10586122665984732, -20.42344490663941414, 35.00000000000000000 ) ) ;
#10858=CLOSED_SHELL ( 'NONE', ( #10468, #12445, #3740, #2458, #12108, #1481, #9447, #7884, #6667, #11504, #13114, #4253, #11327, #8194, #6401, #13743, #3350, #7979, #6712, #4729, #12888, #3922, #7613, #9974, #7904, #1911, #13975, #7248, #2279, #11178, #9419, #10540, #1459, #2718, #1218, #6557, #2954, #7968, #2683, #8859, #8511, #8417, #4379, #3441, #4042, #3158, #370, #6119, #6744, #10762, #1576, #5052, #13265, #13593 ) ) ;
#10862=ORIENTED_EDGE ( 'NONE', *, *, #1266, .T. ) ;
#10884=CARTESIAN_POINT ( 'NONE',  ( 42.20372226782770753, 81.49287499273339108, -25.00000000000000000 ) ) ;
#10894=DIRECTION ( 'NONE',  ( 1.000000000000000000, 0.000000000000000000, 0.000000000000000000 ) ) ;
#10905=PLANE ( 'NONE',  #9762 ) ;
#10917=DIRECTION ( 'NONE',  ( 0.000000000000000000, 0.000000000000000000, -1.000000000000000000 ) ) ;
#10922=DIRECTION ( 'NONE',  ( -1.000000000000000000, 0.000000000000000000, 0.000000000000000000 ) ) ;
#10925=ORIENTED_EDGE ( 'NONE', *, *, #4568, .T. ) ;
#10927=FACE_BOUND ( 'NONE', #12077, .T. ) ;
#10932=CIRCLE ( 'NONE', #4636, 2.500000000000002220 ) ;
#10939=CYLINDRICAL_SURFACE ( 'NONE', #12812, 2.500000000000002220 ) ;
#10943=SURFACE_STYLE_FILL_AREA ( #13381 ) ;
#10951=EDGE_LOOP ( 'NONE', ( #2884, #11146 ) ) ;
#10954=VERTEX_POINT ( 'NONE', #13982 ) ;
#10957=LINE ( 'NONE', #1897, #12378 ) ;
#10965=AXIS2_PLACEMENT_3D ( 'NONE', #11100, #11320, #5535 ) ;
#10966=EDGE_LOOP ( 'NONE', ( #7462, #11059, #14247, #8714 ) ) ;
#10980=CARTESIAN_POINT ( 'NONE',  ( 59.10657227073432551, 3.881474981106830313, -25.00000000000000000 ) ) ;
#10981=DIRECTION ( 'NONE',  ( -0.000000000000000000, -0.000000000000000000, -1.000000000000000000 ) ) ;
#10983=CYLINDRICAL_SURFACE ( 'NONE', #6785, 2.500000000000002220 ) ;
#10984=CARTESIAN_POINT ( 'NONE',  ( 61.68121602037100359, 13.58289998256015352, 25.00000000000000000 ) ) ;
#10986=DIRECTION ( 'NONE',  ( 1.000000000000000000, 0.000000000000000000, 0.000000000000000000 ) ) ;
#10995=AXIS2_PLACEMENT_3D ( 'NONE', #1931, #12992, #10849 ) ;
#10997=CARTESIAN_POINT ( 'NONE',  ( 30.07694101601105530, 130.0000000000000000, -25.00000000000000000 ) ) ;
#10998=VECTOR ( 'NONE', #2557, 1000.000000000000000 ) ;
#10999=FACE_BOUND ( 'NONE', #8494, .T. ) ;
#11002=VERTEX_POINT ( 'NONE', #7379 ) ;
#11010=LINE ( 'NONE', #7568, #8833 ) ;
#11015=EDGE_CURVE ( 'NONE', #10016, #908, #4895, .T. ) ;
#11025=AXIS2_PLACEMENT_3D ( 'NONE', #167, #6524, #5441 ) ;
#11046=EDGE_CURVE ( 'NONE', #55, #908, #10304, .T. ) ;
#11056=EDGE_CURVE ( 'NONE', #3991, #4075, #1199, .T. ) ;
#11059=ORIENTED_EDGE ( 'NONE', *, *, #4900, .T. ) ;
#11060=DIRECTION ( 'NONE',  ( -0.2425356250363329969, 0.9701425001453318764, 9.251858538542973800E-15 ) ) ;
#11061=LINE ( 'NONE', #14291, #7520 ) ;
#11077=EDGE_LOOP ( 'NONE', ( #13757, #12603, #2860, #7162 ) ) ;
#11079=VECTOR ( 'NONE', #8152, 999.9999999999998863 ) ;
#11083=EDGE_CURVE ( 'NONE', #13714, #3050, #3666, .T. ) ;
#11088=CARTESIAN_POINT ( 'NONE',  ( 62.10586122665984732, -20.42344490663941414, -35.00000000000000000 ) ) ;
#11097=ORIENTED_EDGE ( 'NONE', *, *, #5284, .T. ) ;
#11100=CARTESIAN_POINT ( 'NONE',  ( 44.62907851819101523, 71.79144999128007498, 25.00000000000000000 ) ) ;
#11123=CARTESIAN_POINT ( 'NONE',  ( 71.80728622811317052, -17.99808865627607801, -28.00000000000000000 ) ) ;
#11130=DIRECTION ( 'NONE',  ( -1.000000000000000000, 0.000000000000000000, 0.000000000000000000 ) ) ;
#11140=CIRCLE ( 'NONE', #9977, 2.500000000000002220 ) ;
#11146=ORIENTED_EDGE ( 'NONE', *, *, #4337, .T. ) ;
#11156=ORIENTED_EDGE ( 'NONE', *, *, #14256, .T. ) ;
#11170=CARTESIAN_POINT ( 'NONE',  ( 62.10586122665984732, -20.42344490663941414, -25.00000000000000000 ) ) ;
#11171=FACE_OUTER_BOUND ( 'NONE', #5017, .T. ) ;
#11172=DIRECTION ( 'NONE',  ( 0.2425356250363327471, -0.9701425001453319874, -0.000000000000000000 ) ) ;
#11175=CARTESIAN_POINT ( 'NONE',  ( 21.68170757442808849, 141.2731697022877313, 35.00000000000000000 ) ) ;
#11177=CARTESIAN_POINT ( 'NONE',  ( 61.60657227073433262, 3.881474981106830313, 25.00000000000000000 ) ) ;
#11178=ADVANCED_FACE ( 'NONE', ( #13916 ), #5826, .T. ) ;
#11180=ORIENTED_EDGE ( 'NONE', *, *, #14256, .F. ) ;
#11190=DIRECTION ( 'NONE',  ( -1.000000000000000000, 0.000000000000000000, 0.000000000000000000 ) ) ;
#11196=EDGE_CURVE ( 'NONE', #11484, #12547, #1378, .T. ) ;
#11203=CARTESIAN_POINT ( 'NONE',  ( 46.97979101891770171, 52.38859998837343568, -25.00000000000000000 ) ) ;
#11205=DIRECTION ( 'NONE',  ( -0.000000000000000000, -0.000000000000000000, -1.000000000000000000 ) ) ;
#11210=ORIENTED_EDGE ( 'NONE', *, *, #2503, .T. ) ;
#11215=ORIENTED_EDGE ( 'NONE', *, *, #5769, .T. ) ;
#11228=CARTESIAN_POINT ( 'NONE',  ( 61.60657227073433262, 3.881474981106830313, -25.00000000000000000 ) ) ;
#11258=FACE_BOUND ( 'NONE', #12276, .T. ) ;
#11276=EDGE_LOOP ( 'NONE', ( #9456, #4440, #8504, #12940 ) ) ;
#11287=DIRECTION ( 'NONE',  ( 0.000000000000000000, 0.000000000000000000, -1.000000000000000000 ) ) ;
#11290=VECTOR ( 'NONE', #10260, 1000.000000000000000 ) ;
#11291=DIRECTION ( 'NONE',  ( 0.000000000000000000, 0.000000000000000000, -1.000000000000000000 ) ) ;
#11307=DIRECTION ( 'NONE',  ( -0.000000000000000000, -0.000000000000000000, -1.000000000000000000 ) ) ;
#11312=ORIENTED_EDGE ( 'NONE', *, *, #4677, .F. ) ;
#11320=DIRECTION ( 'NONE',  ( 0.000000000000000000, 0.000000000000000000, -1.000000000000000000 ) ) ;
#11327=ADVANCED_FACE ( 'NONE', ( #4038 ), #7445, .T. ) ;
#11330=LINE ( 'NONE', #1300, #8015 ) ;
#11343=CARTESIAN_POINT ( 'NONE',  ( 54.33050351964436686, 32.98574998546678927, 25.00000000000000000 ) ) ;
#11351=CARTESIAN_POINT ( 'NONE',  ( 21.68170757442806362, 141.2731697022877029, -28.00000000000000000 ) ) ;
#11356=DIRECTION ( 'NONE',  ( 1.000000000000000000, 0.000000000000000000, 0.000000000000000000 ) ) ;
#11363=CIRCLE ( 'NONE', #12771, 2.500000000000002220 ) ;
#11364=DIRECTION ( 'NONE',  ( -0.000000000000000000, -0.000000000000000000, -1.000000000000000000 ) ) ;
#11379=EDGE_LOOP ( 'NONE', ( #13220, #8843 ) ) ;
#11396=AXIS2_PLACEMENT_3D ( 'NONE', #536, #9675, #3900 ) ;
#11403=EDGE_CURVE ( 'NONE', #992, #1210, #2151, .T. ) ;
#11405=EDGE_LOOP ( 'NONE', ( #9021, #7657, #9504, #680 ) ) ;
#11412=ORIENTED_EDGE ( 'NONE', *, *, #2517, .F. ) ;
#11418=EDGE_CURVE ( 'NONE', #14384, #7049, #8905, .T. ) ;
#11420=VECTOR ( 'NONE', #12420, 1000.000000000000114 ) ;
#11428=CIRCLE ( 'NONE', #5131, 2.500000000000002220 ) ;
#11433=FACE_OUTER_BOUND ( 'NONE', #8686, .T. ) ;
#11435=CARTESIAN_POINT ( 'NONE',  ( 49.55443476855437268, 62.09002498982675888, 25.00000000000000000 ) ) ;
#11455=EDGE_CURVE ( 'NONE', #5373, #3729, #9854, .T. ) ;
#11461=LINE ( 'NONE', #13687, #10292 ) ;
#11465=CIRCLE ( 'NONE', #10294, 2.500000000000002220 ) ;
#11473=EDGE_CURVE ( 'NONE', #260, #5068, #2039, .T. ) ;
#11477=DIRECTION ( 'NONE',  ( -1.000000000000000000, 0.000000000000000000, 0.000000000000000000 ) ) ;
#11479=CYLINDRICAL_SURFACE ( 'NONE', #1425, 2.500000000000002220 ) ;
#11480=ORIENTED_EDGE ( 'NONE', *, *, #7715, .F. ) ;
#11484=VERTEX_POINT ( 'NONE', #6485 ) ;
#11490=DIRECTION ( 'NONE',  ( 0.000000000000000000, 0.000000000000000000, -1.000000000000000000 ) ) ;
#11491=COLOUR_RGB ( '', 0.08235294, 0.09019608, 0.10196078) ;
#11500=EDGE_CURVE ( 'NONE', #2949, #7089, #3753, .T. ) ;
#11504=ADVANCED_FACE ( 'NONE', ( #8161 ), #1292, .T. ) ;
#11505=CIRCLE ( 'NONE', #5884, 2.500000000000002220 ) ;
#11510=DIRECTION ( 'NONE',  ( 0.2425356250363329969, -0.9701425001453318764, -0.000000000000000000 ) ) ;
#11520=DIRECTION ( 'NONE',  ( -1.000000000000000000, 0.000000000000000000, 0.000000000000000000 ) ) ;
#11529=FACE_OUTER_BOUND ( 'NONE', #4423, .T. ) ;
#11546=ORIENTED_EDGE ( 'NONE', *, *, #7803, .T. ) ;
#11558=CARTESIAN_POINT ( 'NONE',  ( 30.07694101601105530, 130.0000000000000000, -25.00000000000000000 ) ) ;
#11561=DIRECTION ( 'NONE',  ( 0.000000000000000000, 0.000000000000000000, -1.000000000000000000 ) ) ;
#11582=EDGE_CURVE ( 'NONE', #4769, #10016, #2117, .T. ) ;
#11591=FACE_BOUND ( 'NONE', #14172, .T. ) ;
#11612=CIRCLE ( 'NONE', #9286, 2.500000000000002220 ) ;
#11614=CIRCLE ( 'NONE', #13501, 2.500000000000002220 ) ;
#11622=CARTESIAN_POINT ( 'NONE',  ( 21.68170757442808849, 141.2731697022877313, -23.00000000000000000 ) ) ;
#11646=CARTESIAN_POINT ( 'NONE',  ( 54.40514726928103784, 42.68717498692012668, 25.00000000000000000 ) ) ;
#11676=ORIENTED_EDGE ( 'NONE', *, *, #12017, .F. ) ;
#11682=CYLINDRICAL_SURFACE ( 'NONE', #4257, 2.500000000000002220 ) ;
#11686=MANIFOLD_SOLID_BREP ( 'Mirror2', #10858 ) ;
#11690=EDGE_LOOP ( 'NONE', ( #1251, #6468, #5874, #6457 ) ) ;
#11697=CYLINDRICAL_SURFACE ( 'NONE', #1967, 2.500000000000002220 ) ;
#11699=CARTESIAN_POINT ( 'NONE',  ( 39.77836601746437850, 91.19429999418670718, -25.00000000000000000 ) ) ;
#11714=EDGE_LOOP ( 'NONE', ( #2664, #7767, #6625, #6750 ) ) ;
#11720=AXIS2_PLACEMENT_3D ( 'NONE', #3961, #861, #7380 ) ;
#11721=ORIENTED_EDGE ( 'NONE', *, *, #11046, .T. ) ;
#11736=DIRECTION ( 'NONE',  ( -0.2425356250363330801, 0.9701425001453319874, 0.000000000000000000 ) ) ;
#11745=LINE ( 'NONE', #10571, #9570 ) ;
#11751=CARTESIAN_POINT ( 'NONE',  ( 21.68170757442808849, 141.2731697022877313, -23.00000000000000000 ) ) ;
#11764=CARTESIAN_POINT ( 'NONE',  ( 49.47979101891770171, 52.38859998837343568, -25.00000000000000000 ) ) ;
#11769=DIRECTION ( 'NONE',  ( 0.000000000000000000, 0.000000000000000000, -1.000000000000000000 ) ) ;
#11807=EDGE_CURVE ( 'NONE', #3362, #1210, #2382, .T. ) ;
#11808=ORIENTED_EDGE ( 'NONE', *, *, #11473, .F. ) ;
#11821=EDGE_CURVE ( 'NONE', #4176, #11002, #11465, .T. ) ;
#11822=EDGE_CURVE ( 'NONE', #2838, #11484, #5788, .T. ) ;
#11828=FACE_BOUND ( 'NONE', #9377, .T. ) ;
#11838=ORIENTED_EDGE ( 'NONE', *, *, #13545, .F. ) ;
#11842=CARTESIAN_POINT ( 'NONE',  ( 71.80728622811317052, -17.99808865627607801, -25.00000000000000000 ) ) ;
#11845=CARTESIAN_POINT ( 'NONE',  ( 59.10586122665984732, -20.42344490663941414, -35.00000000000000000 ) ) ;
#11867=CARTESIAN_POINT ( 'NONE',  ( 34.85300976710104948, 100.8957249956400375, 25.00000000000000000 ) ) ;
#11868=ORIENTED_EDGE ( 'NONE', *, *, #13259, .T. ) ;
#11893=DIRECTION ( 'NONE',  ( 0.000000000000000000, 0.000000000000000000, -1.000000000000000000 ) ) ;
#11916=VERTEX_POINT ( 'NONE', #2906 ) ;
#11936=EDGE_CURVE ( 'NONE', #7049, #3245, #1640, .T. ) ;
#11937=VERTEX_POINT ( 'NONE', #7114 ) ;
#11947=AXIS2_PLACEMENT_3D ( 'NONE', #9265, #5810, #10289 ) ;
#11953=CARTESIAN_POINT ( 'NONE',  ( 42.12907851819100813, 71.79144999128007498, -25.00000000000000000 ) ) ;
#11954=CARTESIAN_POINT ( 'NONE',  ( 32.50229726637438432, 120.2985749985466839, 25.00000000000000000 ) ) ;
#11957=VECTOR ( 'NONE', #729, 1000.000000000000000 ) ;
#11960=CARTESIAN_POINT ( 'NONE',  ( 34.92765351673772045, 110.5971499970933536, -25.00000000000000000 ) ) ;
#11967=EDGE_CURVE ( 'NONE', #13907, #5068, #13554, .T. ) ;
#11981=DIRECTION ( 'NONE',  ( 0.9701425001453318764, 0.2425356250363329969, 0.000000000000000000 ) ) ;
#12006=AXIS2_PLACEMENT_3D ( 'NONE', #7460, #4136, #5212 ) ;
#12015=LINE ( 'NONE', #3, #8476 ) ;
#12017=EDGE_CURVE ( 'NONE', #8916, #5618, #3526, .T. ) ;
#12035=CARTESIAN_POINT ( 'NONE',  ( 42.27836601746437850, 91.19429999418670718, 25.00000000000000000 ) ) ;
#12044=EDGE_LOOP ( 'NONE', ( #4049, #8477, #1197, #3632 ) ) ;
#12049=ORIENTED_EDGE ( 'NONE', *, *, #141, .F. ) ;
#12051=CARTESIAN_POINT ( 'NONE',  ( 37.27836601746437850, 91.19429999418670718, 25.00000000000000000 ) ) ;
#12053=FACE_OUTER_BOUND ( 'NONE', #2886, .T. ) ;
#12077=EDGE_LOOP ( 'NONE', ( #11180, #6568 ) ) ;
#12078=VECTOR ( 'NONE', #12314, 1000.000000000000000 ) ;
#12086=DIRECTION ( 'NONE',  ( 0.000000000000000000, 0.000000000000000000, -1.000000000000000000 ) ) ;
#12090=AXIS2_PLACEMENT_3D ( 'NONE', #12948, #8233, #2844 ) ;
#12091=DIRECTION ( 'NONE',  ( -1.000000000000000000, 0.000000000000000000, 0.000000000000000000 ) ) ;
#12095=LINE ( 'NONE', #7838, #12078 ) ;
#12096=EDGE_CURVE ( 'NONE', #10101, #6127, #4422, .T. ) ;
#12106=EDGE_LOOP ( 'NONE', ( #4555, #13214, #9233, #5848 ) ) ;
#12108=ADVANCED_FACE ( 'NONE', ( #2563 ), #11479, .T. ) ;
#12109=FACE_BOUND ( 'NONE', #332, .T. ) ;
#12124=APPLICATION_CONTEXT ( 'automotive_design' ) ;
#12126=VERTEX_POINT ( 'NONE', #8186 ) ;
#12130=LINE ( 'NONE', #10143, #6525 ) ;
#12131=DIRECTION ( 'NONE',  ( 0.000000000000000000, 0.000000000000000000, -1.000000000000000000 ) ) ;
#12161=AXIS2_PLACEMENT_3D ( 'NONE', #8236, #8468, #13021 ) ;
#12163=FACE_OUTER_BOUND ( 'NONE', #6012, .T. ) ;
#12188=DIRECTION ( 'NONE',  ( -0.000000000000000000, -0.000000000000000000, -1.000000000000000000 ) ) ;
#12221=VECTOR ( 'NONE', #4892, 1000.000000000000000 ) ;
#12222=EDGE_LOOP ( 'NONE', ( #8689, #2935, #1208, #5764 ) ) ;
#12231=AXIS2_PLACEMENT_3D ( 'NONE', #2330, #483, #12767 ) ;
#12252=VERTEX_POINT ( 'NONE', #9442 ) ;
#12261=DIRECTION ( 'NONE',  ( -1.000000000000000000, 0.000000000000000000, 0.000000000000000000 ) ) ;
#12276=EDGE_LOOP ( 'NONE', ( #10565, #7954 ) ) ;
#12278=EDGE_CURVE ( 'NONE', #13075, #13851, #13838, .T. ) ;
#12281=DIRECTION ( 'NONE',  ( 0.000000000000000000, 0.000000000000000000, 1.000000000000000000 ) ) ;
#12288=VERTEX_POINT ( 'NONE', #6424 ) ;
#12291=EDGE_CURVE ( 'NONE', #7600, #2673, #2602, .T. ) ;
#12310=CARTESIAN_POINT ( 'NONE',  ( 34.92765351673772045, 110.5971499970933536, 25.00000000000000000 ) ) ;
#12314=DIRECTION ( 'NONE',  ( 0.000000000000000000, 0.000000000000000000, -1.000000000000000000 ) ) ;
#12321=CIRCLE ( 'NONE', #12090, 2.500000000000002220 ) ;
#12343=ORIENTED_EDGE ( 'NONE', *, *, #12937, .F. ) ;
#12344=EDGE_LOOP ( 'NONE', ( #2627, #9111, #2553, #14084 ) ) ;
#12351=PLANE ( 'NONE',  #10037 ) ;
#12354=ORIENTED_EDGE ( 'NONE', *, *, #11821, .T. ) ;
#12361=FACE_OUTER_BOUND ( 'NONE', #3589, .T. ) ;
#12378=VECTOR ( 'NONE', #5397, 1000.000000000000000 ) ;
#12382=CIRCLE ( 'NONE', #1389, 2.500000000000002220 ) ;
#12391=VECTOR ( 'NONE', #9611, 1000.000000000000000 ) ;
#12401=CARTESIAN_POINT ( 'NONE',  ( 44.62907851819101523, 71.79144999128007498, 25.00000000000000000 ) ) ;
#12402=EDGE_CURVE ( 'NONE', #3420, #12252, #50, .T. ) ;
#12403=CARTESIAN_POINT ( 'NONE',  ( 39.77836601746437850, 91.19429999418670718, 25.00000000000000000 ) ) ;
#12410=AXIS2_PLACEMENT_3D ( 'NONE', #3518, #6872, #11981 ) ;
#12414=ORIENTED_EDGE ( 'NONE', *, *, #12914, .T. ) ;
#12420=DIRECTION ( 'NONE',  ( -0.2425356250363330524, 0.9701425001453318764, 0.000000000000000000 ) ) ;
#12445=ADVANCED_FACE ( 'NONE', ( #6640 ), #4400, .T. ) ;
#12469=DIRECTION ( 'NONE',  ( 0.000000000000000000, 0.000000000000000000, -1.000000000000000000 ) ) ;
#12476=EDGE_LOOP ( 'NONE', ( #5704, #1149, #8873, #4111 ) ) ;
#12480=DIRECTION ( 'NONE',  ( 0.2425356250363327748, -0.9701425001453319874, -0.000000000000000000 ) ) ;
#12484=ORIENTED_EDGE ( 'NONE', *, *, #7161, .T. ) ;
#12502=ORIENTED_EDGE ( 'NONE', *, *, #4368, .F. ) ;
#12504=ORIENTED_EDGE ( 'NONE', *, *, #11015, .T. ) ;
#12509=ORIENTED_EDGE ( 'NONE', *, *, #3686, .T. ) ;
#12510=CARTESIAN_POINT ( 'NONE',  ( 51.83050351964435976, 32.98574998546678927, 25.00000000000000000 ) ) ;
#12519=VERTEX_POINT ( 'NONE', #13616 ) ;
#12520=ORIENTED_EDGE ( 'NONE', *, *, #11967, .T. ) ;
#12535=VERTEX_POINT ( 'NONE', #7065 ) ;
#12536=CARTESIAN_POINT ( 'NONE',  ( 42.12907851819100813, 71.79144999128007498, 25.00000000000000000 ) ) ;
#12542=CARTESIAN_POINT ( 'NONE',  ( 0.000000000000000000, 0.000000000000000000, 23.00000000000000000 ) ) ;
#12547=VERTEX_POINT ( 'NONE', #4881 ) ;
#12555=DIRECTION ( 'NONE',  ( 0.2425356250363327748, -0.9701425001453319874, -0.000000000000000000 ) ) ;
#12563=VECTOR ( 'NONE', #12710, 1000.000000000000000 ) ;
#12565=DIRECTION ( 'NONE',  ( 0.000000000000000000, 0.000000000000000000, -1.000000000000000000 ) ) ;
#12570=LINE ( 'NONE', #5901, #10998 ) ;
#12573=ORIENTED_EDGE ( 'NONE', *, *, #293, .F. ) ;
#12576=DIRECTION ( 'NONE',  ( -1.000000000000000000, 0.000000000000000000, 0.000000000000000000 ) ) ;
#12582=ORIENTED_EDGE ( 'NONE', *, *, #3829, .T. ) ;
#12584=DIRECTION ( 'NONE',  ( 1.000000000000000000, 0.000000000000000000, 0.000000000000000000 ) ) ;
#12592=CYLINDRICAL_SURFACE ( 'NONE', #554, 2.500000000000002220 ) ;
#12603=ORIENTED_EDGE ( 'NONE', *, *, #13199, .T. ) ;
#12611=FACE_BOUND ( 'NONE', #9083, .T. ) ;
#12618=DIRECTION ( 'NONE',  ( -0.000000000000000000, -0.000000000000000000, -1.000000000000000000 ) ) ;
#12630=VECTOR ( 'NONE', #255, 1000.000000000000000 ) ;
#12635=ORIENTED_EDGE ( 'NONE', *, *, #7522, .F. ) ;
#12637=AXIS2_PLACEMENT_3D ( 'NONE', #11699, #10611, #596 ) ;
#12642=LINE ( 'NONE', #1457, #9646 ) ;
#12660=( GEOMETRIC_REPRESENTATION_CONTEXT ( 3 ) GLOBAL_UNCERTAINTY_ASSIGNED_CONTEXT ( ( #9087 ) ) GLOBAL_UNIT_ASSIGNED_CONTEXT ( ( #2368, #108, #9909 ) ) REPRESENTATION_CONTEXT ( 'NONE', 'WORKASPACE' ) );
#12664=ORIENTED_EDGE ( 'NONE', *, *, #556, .F. ) ;
#12666=CARTESIAN_POINT ( 'NONE',  ( 59.10657227073432551, 3.881474981106830313, 25.00000000000000000 ) ) ;
#12684=EDGE_LOOP ( 'NONE', ( #2104, #10495, #6956, #10018 ) ) ;
#12690=EDGE_LOOP ( 'NONE', ( #3332, #11210, #1452, #2938 ) ) ;
#12691=DIRECTION ( 'NONE',  ( 0.000000000000000000, 0.000000000000000000, -1.000000000000000000 ) ) ;
#12692=CARTESIAN_POINT ( 'NONE',  ( 21.68170757442808849, 141.2731697022877313, 23.00000000000000000 ) ) ;
#12700=LINE ( 'NONE', #9562, #11079 ) ;
#12701=CARTESIAN_POINT ( 'NONE',  ( 18.68170757442808849, 141.2731697022877313, 35.00000000000000000 ) ) ;
#12709=DIRECTION ( 'NONE',  ( -1.000000000000000000, 0.000000000000000000, 0.000000000000000000 ) ) ;
#12710=DIRECTION ( 'NONE',  ( 0.000000000000000000, 0.000000000000000000, -1.000000000000000000 ) ) ;
#12716=EDGE_CURVE ( 'NONE', #12827, #13075, #9062, .T. ) ;
#12720=EDGE_CURVE ( 'NONE', #13907, #5618, #3236, .T. ) ;
#12738=LINE ( 'NONE', #7018, #2473 ) ;
#12741=ORIENTED_EDGE ( 'NONE', *, *, #10484, .T. ) ;
#12753=LINE ( 'NONE', #1789, #12391 ) ;
#12757=DIRECTION ( 'NONE',  ( 0.000000000000000000, 0.000000000000000000, -1.000000000000000000 ) ) ;
#12767=DIRECTION ( 'NONE',  ( 1.000000000000000000, 0.000000000000000000, 0.000000000000000000 ) ) ;
#12771=AXIS2_PLACEMENT_3D ( 'NONE', #6516, #6595, #3401 ) ;
#12775=DIRECTION ( 'NONE',  ( 1.000000000000000000, 0.000000000000000000, 0.000000000000000000 ) ) ;
#12784=AXIS2_PLACEMENT_3D ( 'NONE', #2824, #3694, #1719 ) ;
#12787=VECTOR ( 'NONE', #5298, 999.9999999999998863 ) ;
#12808=CIRCLE ( 'NONE', #7428, 2.500000000000002220 ) ;
#12812=AXIS2_PLACEMENT_3D ( 'NONE', #911, #5379, #2447 ) ;
#12827=VERTEX_POINT ( 'NONE', #12666 ) ;
#12888=ADVANCED_FACE ( 'NONE', ( #7026 ), #1549, .F. ) ;
#12897=DIRECTION ( 'NONE',  ( -0.2425356250363327748, 0.9701425001453319874, 0.000000000000000000 ) ) ;
#12901=ORIENTED_EDGE ( 'NONE', *, *, #2982, .T. ) ;
#12912=AXIS2_PLACEMENT_3D ( 'NONE', #6299, #13054, #1849 ) ;
#12914=EDGE_CURVE ( 'NONE', #2673, #7600, #8913, .T. ) ;
#12917=FACE_OUTER_BOUND ( 'NONE', #2807, .T. ) ;
#12931=VECTOR ( 'NONE', #8041, 1000.000000000000000 ) ;
#12937=EDGE_CURVE ( 'NONE', #4466, #1176, #5282, .T. ) ;
#12938=CARTESIAN_POINT ( 'NONE',  ( 51.90514726928103073, 42.68717498692012668, 25.00000000000000000 ) ) ;
#12940=ORIENTED_EDGE ( 'NONE', *, *, #12720, .T. ) ;
#12948=CARTESIAN_POINT ( 'NONE',  ( 47.05443476855437268, 62.09002498982675888, 25.00000000000000000 ) ) ;
#12950=DIRECTION ( 'NONE',  ( 0.000000000000000000, 0.000000000000000000, -1.000000000000000000 ) ) ;
#12981=ORIENTED_EDGE ( 'NONE', *, *, #3243, .T. ) ;
#12992=DIRECTION ( 'NONE',  ( 0.000000000000000000, 0.000000000000000000, -1.000000000000000000 ) ) ;
#12995=ORIENTED_EDGE ( 'NONE', *, *, #12720, .F. ) ;
#13000=CARTESIAN_POINT ( 'NONE',  ( 30.00229726637438432, 120.2985749985466839, 25.00000000000000000 ) ) ;
#13011=VECTOR ( 'NONE', #11736, 999.9999999999998863 ) ;
#13021=DIRECTION ( 'NONE',  ( 1.000000000000000000, 0.000000000000000000, 0.000000000000000000 ) ) ;
#13025=ORIENTED_EDGE ( 'NONE', *, *, #11822, .T. ) ;
#13035=VECTOR ( 'NONE', #2738, 1000.000000000000000 ) ;
#13054=DIRECTION ( 'NONE',  ( -0.000000000000000000, -0.000000000000000000, -1.000000000000000000 ) ) ;
#13059=DIRECTION ( 'NONE',  ( 0.000000000000000000, 0.000000000000000000, -1.000000000000000000 ) ) ;
#13060=DIRECTION ( 'NONE',  ( 0.000000000000000000, 0.000000000000000000, -1.000000000000000000 ) ) ;
#13061=PLANE ( 'NONE',  #9268 ) ;
#13074=DIRECTION ( 'NONE',  ( -0.000000000000000000, -0.000000000000000000, -1.000000000000000000 ) ) ;
#13075=VERTEX_POINT ( 'NONE', #10980 ) ;
#13082=LINE ( 'NONE', #3133, #6816 ) ;
#13083=ORIENTED_EDGE ( 'NONE', *, *, #13856, .F. ) ;
#13086=EDGE_CURVE ( 'NONE', #12252, #10954, #11061, .T. ) ;
#13096=EDGE_LOOP ( 'NONE', ( #3161, #5123 ) ) ;
#13106=CARTESIAN_POINT ( 'NONE',  ( 62.10586122665984732, -20.42344490663941414, 35.00000000000000000 ) ) ;
#13114=ADVANCED_FACE ( 'NONE', ( #10105 ), #6660, .T. ) ;
#13116=DIRECTION ( 'NONE',  ( -1.000000000000000000, 0.000000000000000000, 0.000000000000000000 ) ) ;
#13120=ORIENTED_EDGE ( 'NONE', *, *, #8557, .T. ) ;
#13125=AXIS2_PLACEMENT_3D ( 'NONE', #6022, #566, #6185 ) ;
#13130=CYLINDRICAL_SURFACE ( 'NONE', #2773, 2.500000000000002220 ) ;
#13163=CARTESIAN_POINT ( 'NONE',  ( 18.68170757442808849, 141.2731697022877313, -23.00000000000000000 ) ) ;
#13165=AXIS2_PLACEMENT_3D ( 'NONE', #304, #3824, #11561 ) ;
#13170=FACE_OUTER_BOUND ( 'NONE', #12044, .T. ) ;
#13174=EDGE_LOOP ( 'NONE', ( #13451, #7963, #6713, #1508 ) ) ;
#13188=EDGE_CURVE ( 'NONE', #5967, #8043, #4765, .T. ) ;
#13189=EDGE_CURVE ( 'NONE', #2673, #1985, #8260, .T. ) ;
#13199=EDGE_CURVE ( 'NONE', #8916, #3067, #2644, .T. ) ;
#13212=CARTESIAN_POINT ( 'NONE',  ( 37.35300976710104948, 100.8957249956400375, 25.00000000000000000 ) ) ;
#13214=ORIENTED_EDGE ( 'NONE', *, *, #7682, .T. ) ;
#13219=FACE_BOUND ( 'NONE', #8263, .T. ) ;
#13220=ORIENTED_EDGE ( 'NONE', *, *, #3247, .T. ) ;
#13231=SURFACE_SIDE_STYLE ('',( #10943 ) ) ;
#13234=VECTOR ( 'NONE', #3608, 999.9999999999998863 ) ;
#13237=DIRECTION ( 'NONE',  ( 0.000000000000000000, 0.000000000000000000, -1.000000000000000000 ) ) ;
#13249=CARTESIAN_POINT ( 'NONE',  ( 30.00229726637438432, 120.2985749985466839, 25.00000000000000000 ) ) ;
#13253=CIRCLE ( 'NONE', #6924, 2.500000000000002220 ) ;
#13259=EDGE_CURVE ( 'NONE', #12519, #1702, #4056, .T. ) ;
#13265=ADVANCED_FACE ( 'NONE', ( #4902 ), #4627, .F. ) ;
#13274=DIRECTION ( 'NONE',  ( -0.000000000000000000, -0.000000000000000000, -1.000000000000000000 ) ) ;
#13295=DIRECTION ( 'NONE',  ( 1.000000000000000000, 0.000000000000000000, 0.000000000000000000 ) ) ;
#13297=FACE_OUTER_BOUND ( 'NONE', #2393, .T. ) ;
#13299=SURFACE_STYLE_USAGE ( .BOTH. , #13231 ) ;
#13324=EDGE_CURVE ( 'NONE', #13714, #6682, #5196, .T. ) ;
#13325=EDGE_CURVE ( 'NONE', #2033, #12126, #8408, .T. ) ;
#13326=VECTOR ( 'NONE', #8638, 1000.000000000000114 ) ;
#13331=FACE_OUTER_BOUND ( 'NONE', #10966, .T. ) ;
#13363=SURFACE_STYLE_FILL_AREA ( #4365 ) ;
#13375=EDGE_CURVE ( 'NONE', #1702, #12519, #1700, .T. ) ;
#13381=FILL_AREA_STYLE ('',( #7718 ) ) ;
#13396=CARTESIAN_POINT ( 'NONE',  ( 71.80728622811317052, -17.99808865627607801, 28.00000000000000000 ) ) ;
#13406=AXIS2_PLACEMENT_3D ( 'NONE', #4129, #1917, #5201 ) ;
#13409=LINE ( 'NONE', #6427, #5476 ) ;
#13412=DIRECTION ( 'NONE',  ( 0.000000000000000000, 0.000000000000000000, -1.000000000000000000 ) ) ;
#13418=DIRECTION ( 'NONE',  ( 0.000000000000000000, 0.000000000000000000, -1.000000000000000000 ) ) ;
#13426=CARTESIAN_POINT ( 'NONE',  ( 39.77836601746437850, 91.19429999418670718, 25.00000000000000000 ) ) ;
#13428=EDGE_LOOP ( 'NONE', ( #12981, #3189, #10612, #14191 ) ) ;
#13431=VECTOR ( 'NONE', #8614, 999.9999999999998863 ) ;
#13441=EDGE_LOOP ( 'NONE', ( #12664, #12741, #6966, #9621 ) ) ;
#13449=( LENGTH_UNIT ( ) NAMED_UNIT ( * ) SI_UNIT ( .MILLI., .METRE. ) );
#13451=ORIENTED_EDGE ( 'NONE', *, *, #9520, .F. ) ;
#13461=CARTESIAN_POINT ( 'NONE',  ( 49.40514726928103073, 42.68717498692012668, 25.00000000000000000 ) ) ;
#13464=CARTESIAN_POINT ( 'NONE',  ( 32.50229726637438432, 120.2985749985466839, -25.00000000000000000 ) ) ;
#13495=CARTESIAN_POINT ( 'NONE',  ( 71.80728622811317052, -17.99808865627607801, -28.00000000000000000 ) ) ;
#13496=DIRECTION ( 'NONE',  ( -1.000000000000000000, 0.000000000000000000, 0.000000000000000000 ) ) ;
#13497=ORIENTED_EDGE ( 'NONE', *, *, #13733, .T. ) ;
#13501=AXIS2_PLACEMENT_3D ( 'NONE', #11764, #648, #9261 ) ;
#13515=CARTESIAN_POINT ( 'NONE',  ( 21.68170757442808849, 141.2731697022877313, 23.00000000000000000 ) ) ;
#13532=AXIS2_PLACEMENT_3D ( 'NONE', #12403, #2380, #2903 ) ;
#13539=VERTEX_POINT ( 'NONE', #13249 ) ;
#13545=EDGE_CURVE ( 'NONE', #11937, #1484, #7815, .T. ) ;
#13548=CARTESIAN_POINT ( 'NONE',  ( 62.10586122665987574, -20.42344490663940704, 25.00000000000000000 ) ) ;
#13552=DIRECTION ( 'NONE',  ( 0.000000000000000000, 0.000000000000000000, -1.000000000000000000 ) ) ;
#13554=LINE ( 'NONE', #219, #2373 ) ;
#13569=ORIENTED_EDGE ( 'NONE', *, *, #6189, .T. ) ;
#13570=CYLINDRICAL_SURFACE ( 'NONE', #4179, 2.500000000000002220 ) ;
#13574=VERTEX_POINT ( 'NONE', #12692 ) ;
#13587=VECTOR ( 'NONE', #10780, 1000.000000000000000 ) ;
#13591=CARTESIAN_POINT ( 'NONE',  ( 47.05443476855437268, 62.09002498982675888, 25.00000000000000000 ) ) ;
#13593=ADVANCED_FACE ( 'NONE', ( #10578, #2833, #11258, #12611, #6786, #564, #8293, #5019, #6183, #1569, #1648, #2756, #5081, #11591, #7882, #12361 ), #5946, .F. ) ;
#13604=ORIENTED_EDGE ( 'NONE', *, *, #141, .T. ) ;
#13616=CARTESIAN_POINT ( 'NONE',  ( 39.85300976710104948, 100.8957249956400375, 25.00000000000000000 ) ) ;
#13618=CIRCLE ( 'NONE', #1449, 2.500000000000002220 ) ;
#13622=ORIENTED_EDGE ( 'NONE', *, *, #2392, .F. ) ;
#13629=DIRECTION ( 'NONE',  ( -0.9701425001453318764, -0.2425356250363329969, 0.000000000000000000 ) ) ;
#13638=CARTESIAN_POINT ( 'NONE',  ( 71.80728622811317052, -17.99808865627607801, -25.00000000000000000 ) ) ;
#13656=UNCERTAINTY_MEASURE_WITH_UNIT (LENGTH_MEASURE( 1.000000000000000082E-05 ), #13449, 'distance_accuracy_value', 'NONE');
#13676=DIRECTION ( 'NONE',  ( 0.000000000000000000, 1.000000000000000000, 0.000000000000000000 ) ) ;
#13683=DIRECTION ( 'NONE',  ( -0.000000000000000000, -0.000000000000000000, -1.000000000000000000 ) ) ;
#13687=CARTESIAN_POINT ( 'NONE',  ( 59.10586122665984732, -20.42344490663941414, 35.00000000000000000 ) ) ;
#13692=CARTESIAN_POINT ( 'NONE',  ( 31.38313257588138683, 143.6985259526510390, 28.00000000000000000 ) ) ;
#13705=ORIENTED_EDGE ( 'NONE', *, *, #12291, .F. ) ;
#13714=VERTEX_POINT ( 'NONE', #5444 ) ;
#13729=AXIS2_PLACEMENT_3D ( 'NONE', #4835, #2651, #5701 ) ;
#13733=EDGE_CURVE ( 'NONE', #11916, #7552, #14332, .T. ) ;
#13739=EDGE_LOOP ( 'NONE', ( #5275, #7250 ) ) ;
#13743=ADVANCED_FACE ( 'NONE', ( #707, #8665, #10927, #901, #13219, #5371, #9914, #9834, #3191, #7619, #12109, #2913, #10999, #7352, #11828, #1801 ), #4091, .F. ) ;
#13744=CARTESIAN_POINT ( 'NONE',  ( 51.97979101891770171, 52.38859998837343568, 25.00000000000000000 ) ) ;
#13749=DIRECTION ( 'NONE',  ( 0.2425356250363327748, -0.9701425001453319874, -0.000000000000000000 ) ) ;
#13757=ORIENTED_EDGE ( 'NONE', *, *, #2348, .F. ) ;
#13760=CIRCLE ( 'NONE', #11396, 2.500000000000002220 ) ;
#13763=DIRECTION ( 'NONE',  ( 0.000000000000000000, 0.000000000000000000, -1.000000000000000000 ) ) ;
#13764=LINE ( 'NONE', #8174, #12221 ) ;
#13791=EDGE_LOOP ( 'NONE', ( #10126, #899, #8982, #829, #4443, #10790 ) ) ;
#13803=CARTESIAN_POINT ( 'NONE',  ( 71.80728622811317052, -17.99808865627607801, 25.00000000000000000 ) ) ;
#13808=ORIENTED_EDGE ( 'NONE', *, *, #12278, .T. ) ;
#13819=DIRECTION ( 'NONE',  ( -1.000000000000000000, 0.000000000000000000, 0.000000000000000000 ) ) ;
#13827=CARTESIAN_POINT ( 'NONE',  ( 32.57694101601105530, 130.0000000000000000, 25.00000000000000000 ) ) ;
#13838=CIRCLE ( 'NONE', #5411, 2.500000000000002220 ) ;
#13841=DIRECTION ( 'NONE',  ( 0.000000000000000000, 0.000000000000000000, -1.000000000000000000 ) ) ;
#13842=EDGE_CURVE ( 'NONE', #2603, #8545, #1125, .T. ) ;
#13851=VERTEX_POINT ( 'NONE', #2370 ) ;
#13856=EDGE_CURVE ( 'NONE', #1484, #3708, #8934, .T. ) ;
#13857=AXIS2_PLACEMENT_3D ( 'NONE', #13426, #12086, #11130 ) ;
#13861=ORIENTED_EDGE ( 'NONE', *, *, #5769, .F. ) ;
#13871=LINE ( 'NONE', #8057, #11290 ) ;
#13874=CARTESIAN_POINT ( 'NONE',  ( 37.35300976710104948, 100.8957249956400375, -25.00000000000000000 ) ) ;
#13876=DIRECTION ( 'NONE',  ( -0.000000000000000000, -0.000000000000000000, -1.000000000000000000 ) ) ;
#13881=AXIS2_PLACEMENT_3D ( 'NONE', #10208, #2318, #8009 ) ;
#13882=EDGE_LOOP ( 'NONE', ( #11412, #403 ) ) ;
#13891=CARTESIAN_POINT ( 'NONE',  ( 37.42765351673772045, 110.5971499970933536, 25.00000000000000000 ) ) ;
#13907=VERTEX_POINT ( 'NONE', #5000 ) ;
#13916=FACE_OUTER_BOUND ( 'NONE', #8897, .T. ) ;
#13923=EDGE_LOOP ( 'NONE', ( #3028, #1703, #8492, #474, #8527, #14028 ) ) ;
#13930=ORIENTED_EDGE ( 'NONE', *, *, #2914, .F. ) ;
#13934=LINE ( 'NONE', #8350, #13587 ) ;
#13936=CARTESIAN_POINT ( 'NONE',  ( 51.90514726928103073, 42.68717498692012668, -25.00000000000000000 ) ) ;
#13939=DIRECTION ( 'NONE',  ( 0.000000000000000000, 0.000000000000000000, -1.000000000000000000 ) ) ;
#13942=FACE_OUTER_BOUND ( 'NONE', #13923, .T. ) ;
#13960=DIRECTION ( 'NONE',  ( 0.000000000000000000, 0.000000000000000000, -1.000000000000000000 ) ) ;
#13964=DIRECTION ( 'NONE',  ( 0.000000000000000000, 0.000000000000000000, -1.000000000000000000 ) ) ;
#13975=ADVANCED_FACE ( 'NONE', ( #2505 ), #12592, .T. ) ;
#13982=CARTESIAN_POINT ( 'NONE',  ( 32.42765351673771335, 110.5971499970933536, -25.00000000000000000 ) ) ;
#13997=CIRCLE ( 'NONE', #10463, 2.500000000000002220 ) ;
#14000=AXIS2_PLACEMENT_3D ( 'NONE', #13874, #12757, #1638 ) ;
#14002=EDGE_LOOP ( 'NONE', ( #3057, #6683 ) ) ;
#14007=ORIENTED_EDGE ( 'NONE', *, *, #3267, .F. ) ;
#14014=VECTOR ( 'NONE', #12480, 999.9999999999998863 ) ;
#14027=EDGE_LOOP ( 'NONE', ( #10381, #9293, #7865, #8804 ) ) ;
#14028=ORIENTED_EDGE ( 'NONE', *, *, #6989, .F. ) ;
#14053=AXIS2_PLACEMENT_3D ( 'NONE', #5808, #6988, #9113 ) ;
#14066=PRODUCT_CONTEXT ( 'NONE', #12124, 'mechanical' ) ;
#14072=VECTOR ( 'NONE', #6879, 1000.000000000000114 ) ;
#14074=DIRECTION ( 'NONE',  ( -0.9701425001453319874, -0.2425356250363328026, 0.000000000000000000 ) ) ;
#14078=VECTOR ( 'NONE', #9940, 1000.000000000000000 ) ;
#14084=ORIENTED_EDGE ( 'NONE', *, *, #9141, .F. ) ;
#14089=AXIS2_PLACEMENT_3D ( 'NONE', #11343, #1312, #2948 ) ;
#14100=ORIENTED_EDGE ( 'NONE', *, *, #3167, .F. ) ;
#14108=DIRECTION ( 'NONE',  ( 0.000000000000000000, 0.000000000000000000, 1.000000000000000000 ) ) ;
#14125=EDGE_CURVE ( 'NONE', #10954, #4122, #3361, .T. ) ;
#14127=VECTOR ( 'NONE', #14128, 999.9999999999998863 ) ;
#14128=DIRECTION ( 'NONE',  ( -0.2425356250363330801, 0.9701425001453319874, 0.000000000000000000 ) ) ;
#14139=DIRECTION ( 'NONE',  ( -0.000000000000000000, -0.000000000000000000, -1.000000000000000000 ) ) ;
#14140=CIRCLE ( 'NONE', #8259, 2.500000000000002220 ) ;
#14147=DIRECTION ( 'NONE',  ( 0.2425356250363328026, -0.9701425001453319874, -0.000000000000000000 ) ) ;
#14154=EDGE_CURVE ( 'NONE', #12126, #2603, #6436, .T. ) ;
#14164=CARTESIAN_POINT ( 'NONE',  ( 31.38313257588138683, 143.6985259526510674, -25.00000000000000000 ) ) ;
#14172=EDGE_LOOP ( 'NONE', ( #13808, #2497 ) ) ;
#14191=ORIENTED_EDGE ( 'NONE', *, *, #75, .F. ) ;
#14200=VECTOR ( 'NONE', #2902, 1000.000000000000114 ) ;
#14216=DIRECTION ( 'NONE',  ( -0.000000000000000000, -0.000000000000000000, -1.000000000000000000 ) ) ;
#14220=CYLINDRICAL_SURFACE ( 'NONE', #187, 2.500000000000002220 ) ;
#14222=VECTOR ( 'NONE', #7809, 1000.000000000000000 ) ;
#14228=LINE ( 'NONE', #10852, #13035 ) ;
#14229=AXIS2_PLACEMENT_3D ( 'NONE', #6411, #2853, #848 ) ;
#14236=DIRECTION ( 'NONE',  ( -1.000000000000000000, 0.000000000000000000, 0.000000000000000000 ) ) ;
#14240=DIRECTION ( 'NONE',  ( 1.000000000000000000, 0.000000000000000000, 0.000000000000000000 ) ) ;
#14247=ORIENTED_EDGE ( 'NONE', *, *, #9141, .T. ) ;
#14256=EDGE_CURVE ( 'NONE', #12252, #3420, #8943, .T. ) ;
#14262=CARTESIAN_POINT ( 'NONE',  ( 51.90514726928103073, 42.68717498692012668, -25.00000000000000000 ) ) ;
#14270=SHAPE_DEFINITION_REPRESENTATION ( #3823, #852 ) ;
#14277=ORIENTED_EDGE ( 'NONE', *, *, #10625, .F. ) ;
#14286=DIRECTION ( 'NONE',  ( 1.000000000000000000, 0.000000000000000000, 0.000000000000000000 ) ) ;
#14289=CARTESIAN_POINT ( 'NONE',  ( 39.77836601746437850, 91.19429999418670718, 25.00000000000000000 ) ) ;
#14291=CARTESIAN_POINT ( 'NONE',  ( 32.42765351673771335, 110.5971499970933536, 25.00000000000000000 ) ) ;
#14324=DIRECTION ( 'NONE',  ( -0.2425356250363328026, 0.9701425001453319874, 0.000000000000000000 ) ) ;
#14332=CIRCLE ( 'NONE', #7314, 2.500000000000002220 ) ;
#14342=CARTESIAN_POINT ( 'NONE',  ( 44.62907851819101523, 71.79144999128007498, -25.00000000000000000 ) ) ;
#14364=ORIENTED_EDGE ( 'NONE', *, *, #150, .F. ) ;
#14371=PRODUCT_DEFINITION_CONTEXT ( 'detailed design', #552, 'design' ) ;
#14384=VERTEX_POINT ( 'NONE', #1421 ) ;
#14410=PLANE ( 'NONE',  #10746 ) ;
#14421=ORIENTED_EDGE ( 'NONE', *, *, #11822, .F. ) ;
#14434=EDGE_CURVE ( 'NONE', #13539, #192, #13618, .T. ) ;
ENDSEC;
END-ISO-10303-21;
